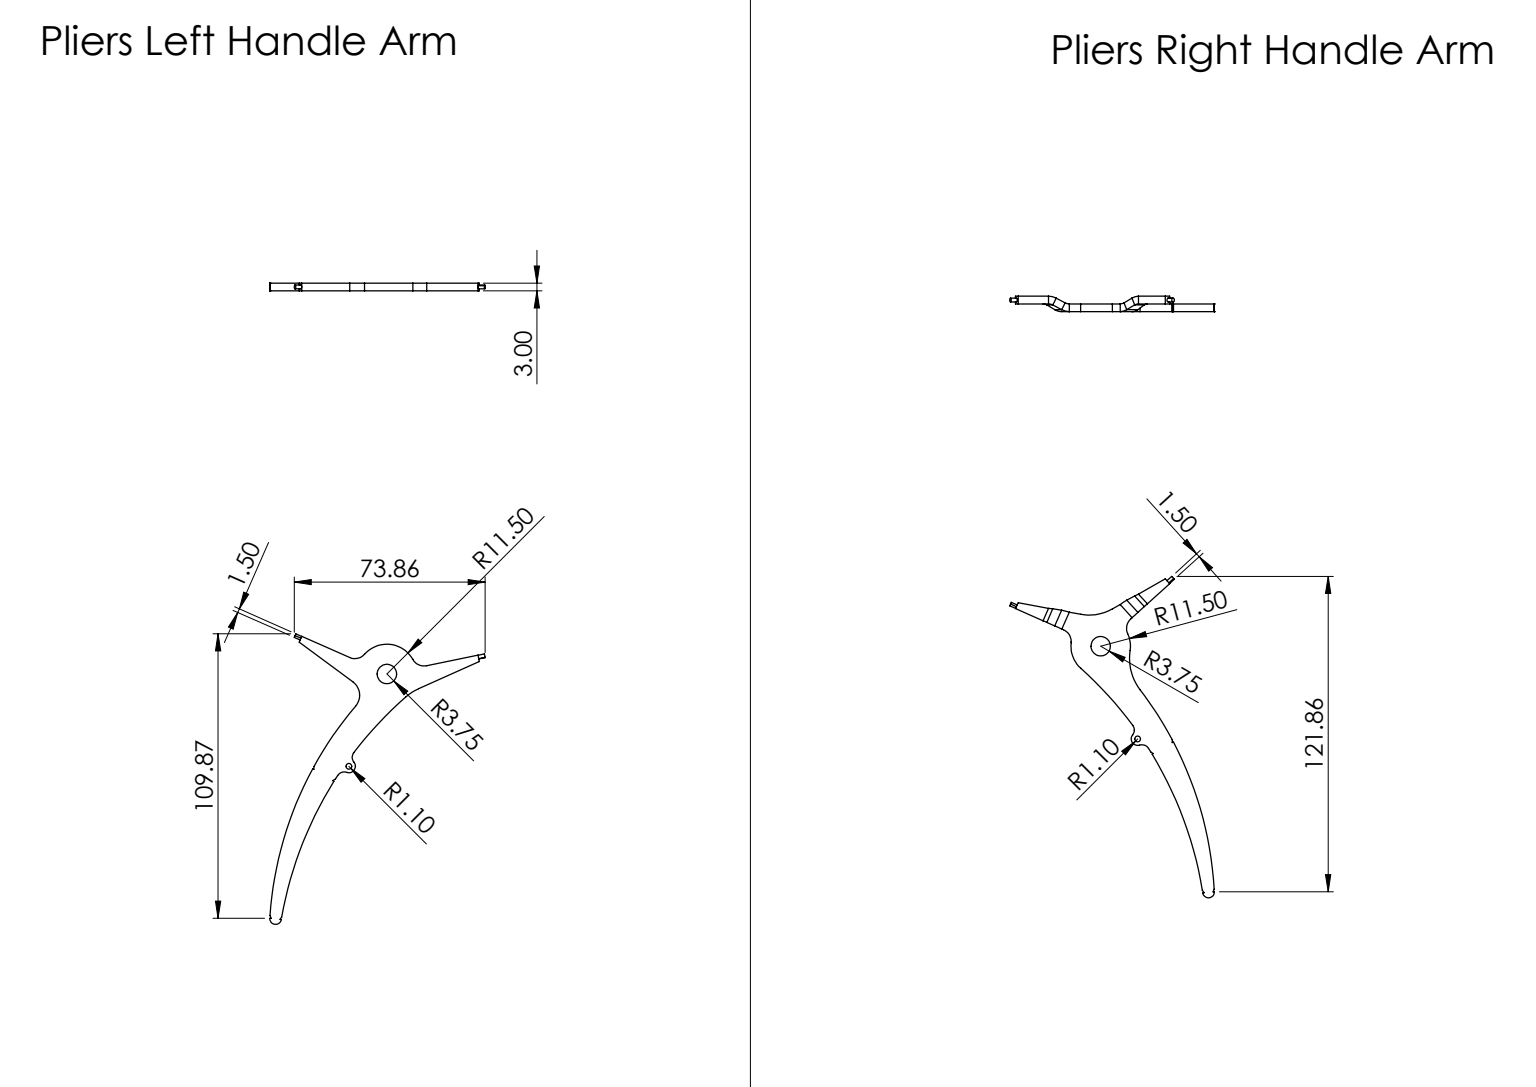
ISO-10303-21;
HEADER;
FILE_DESCRIPTION (('STEP AP214'),
    '1' );
FILE_NAME ('Pliers Right Handle Arm.step',
    '2026-10-09T15:01:35',
    ( '' ),
    ( '' ),
    'SwSTEP 2.0',
    'SolidWorks 2026',
    '' );
FILE_SCHEMA (( 'AUTOMOTIVE_DESIGN' ));
ENDSEC;

DATA;
#2=CIRCLE ( 'NONE', #2039, 3.300000000000002931 ) ;
#5=EDGE_CURVE ( 'NONE', #1930, #3517, #6589, .T. ) ;
#9=CARTESIAN_POINT ( 'NONE',  ( -105.7473861751082040, -118.0666774205683822, -1.188285581044112860E-13 ) ) ;
#10=ORIENTED_EDGE ( 'NONE', *, *, #1499, .F. ) ;
#11=CARTESIAN_POINT ( 'NONE',  ( 39.48483786921892857, -95.33781693134928048, -9.497611030973018842E-14 ) ) ;
#15=EDGE_CURVE ( 'NONE', #320, #2542, #2080, .T. ) ;
#17=CARTESIAN_POINT ( 'NONE',  ( -31.91091272472834817, 16.82560631625344172, 0.006154456448481410852 ) ) ;
#25=AXIS2_PLACEMENT_3D ( 'NONE', #4428, #5501, #4998 ) ;
#26=LINE ( 'NONE', #2324, #1475 ) ;
#28=ADVANCED_FACE ( 'NONE', ( #2146 ), #5063, .T. ) ;
#34=AXIS2_PLACEMENT_3D ( 'NONE', #6184, #972, #7294 ) ;
#35=FACE_OUTER_BOUND ( 'NONE', #4506, .T. ) ;
#37=AXIS2_PLACEMENT_3D ( 'NONE', #1867, #698, #7061 ) ;
#40=AXIS2_PLACEMENT_3D ( 'NONE', #4287, #3708, #845 ) ;
#41=CARTESIAN_POINT ( 'NONE',  ( -7.922926035662746003, 12.41525034409755612, 2.701156757981117984 ) ) ;
#43=FILL_AREA_STYLE_COLOUR ( '', #963 ) ;
#50=AXIS2_PLACEMENT_3D ( 'NONE', #2705, #5732, #561 ) ;
#58=CARTESIAN_POINT ( 'NONE',  ( -15.00216760413269945, 6.625337177075938833, -3.299999999999993161 ) ) ;
#64=CARTESIAN_POINT ( 'NONE',  ( 43.95774332523846795, -95.00278575785266355, -9.454242944073598665E-14 ) ) ;
#68=ADVANCED_FACE ( 'NONE', ( #2687 ), #435, .T. ) ;
#70=VERTEX_POINT ( 'NONE', #2112 ) ;
#75=VERTEX_POINT ( 'NONE', #4424 ) ;
#76=EDGE_CURVE ( 'NONE', #70, #4585, #6096, .T. ) ;
#77=EDGE_CURVE ( 'NONE', #427, #2020, #919, .T. ) ;
#79=CARTESIAN_POINT ( 'NONE',  ( 12.48153656191966476, 18.70005575237079043, -2.479608496603234347 ) ) ;
#81=DIRECTION ( 'NONE',  ( -5.715354789845005112E-18, -9.999836672264339449E-16, 1.000000000000000000 ) ) ;
#89=VERTEX_POINT ( 'NONE', #7308 ) ;
#90=ADVANCED_FACE ( 'NONE', ( #990 ), #3285, .T. ) ;
#92=CARTESIAN_POINT ( 'NONE',  ( 9.769309212388114005, 25.48802373141157673, -2.993845543551514776 ) ) ;
#98=ORIENTED_EDGE ( 'NONE', *, *, #6789, .F. ) ;
#101=PLANE ( 'NONE',  #156 ) ;
#104=EDGE_CURVE ( 'NONE', #5945, #4359, #7121, .T. ) ;
#105=ORIENTED_EDGE ( 'NONE', *, *, #119, .T. ) ;
#106=VERTEX_POINT ( 'NONE', #6746 ) ;
#111=EDGE_CURVE ( 'NONE', #70, #3385, #1232, .T. ) ;
#114=ORIENTED_EDGE ( 'NONE', *, *, #332, .F. ) ;
#117=CARTESIAN_POINT ( 'NONE',  ( -20.16480223318149356, 14.61937842657788345, -2.993845543551524990 ) ) ;
#118=CARTESIAN_POINT ( 'NONE',  ( 9.769309212388092689, 25.48802373141157318, 0.006154456448490518150 ) ) ;
#119=EDGE_CURVE ( 'NONE', #427, #4029, #5685, .T. ) ;
#120=ADVANCED_FACE ( 'NONE', ( #5785 ), #4047, .F. ) ;
#122=AXIS2_PLACEMENT_3D ( 'NONE', #4190, #238, #5631 ) ;
#125=AXIS2_PLACEMENT_3D ( 'NONE', #6895, #3541, #4566 ) ;
#130=ORIENTED_EDGE ( 'NONE', *, *, #2556, .T. ) ;
#138=VERTEX_POINT ( 'NONE', #4690 ) ;
#139=ORIENTED_EDGE ( 'NONE', *, *, #2264, .T. ) ;
#147=CIRCLE ( 'NONE', #6885, 6.299999999999998934 ) ;
#148=AXIS2_PLACEMENT_3D ( 'NONE', #6165, #6059, #1524 ) ;
#150=VECTOR ( 'NONE', #1771, 1000.000000000000227 ) ;
#156=AXIS2_PLACEMENT_3D ( 'NONE', #5801, #629, #4670 ) ;
#161=EDGE_CURVE ( 'NONE', #2317, #4548, #3992, .T. ) ;
#163=LINE ( 'NONE', #7048, #1585 ) ;
#165=CARTESIAN_POINT ( 'NONE',  ( 12.40979888490706706, -30.61452125107581068, 2.999999999999969802 ) ) ;
#174=ORIENTED_EDGE ( 'NONE', *, *, #2963, .T. ) ;
#175=EDGE_CURVE ( 'NONE', #6662, #3589, #2174, .T. ) ;
#178=PLANE ( 'NONE',  #37 ) ;
#184=VERTEX_POINT ( 'NONE', #578 ) ;
#187=CARTESIAN_POINT ( 'NONE',  ( 27.98760434640042050, 26.43260972569849443, -1.493845543551990174 ) ) ;
#190=PLANE ( 'NONE',  #25 ) ;
#191=ORIENTED_EDGE ( 'NONE', *, *, #892, .F. ) ;
#196=PRODUCT ( 'Pliers Right Handle Arm', 'Pliers Right Handle Arm', '', ( #6070 ) ) ;
#198=EDGE_CURVE ( 'NONE', #3368, #5232, #6974, .T. ) ;
#199=ORIENTED_EDGE ( 'NONE', *, *, #978, .F. ) ;
#200=DIRECTION ( 'NONE',  ( 0.9999836672264332815, -0.005715354789844959149, 0.000000000000000000 ) ) ;
#206=EDGE_CURVE ( 'NONE', #2991, #6689, #4958, .T. ) ;
#207=CARTESIAN_POINT ( 'NONE',  ( -17.21006346072928750, 13.86884027412869180, -2.230393353321906247 ) ) ;
#208=ORIENTED_EDGE ( 'NONE', *, *, #252, .F. ) ;
#209=ADVANCED_FACE ( 'NONE', ( #688 ), #379, .F. ) ;
#212=VERTEX_POINT ( 'NONE', #11 ) ;
#213=DIRECTION ( 'NONE',  ( -5.715354789845005112E-18, -9.999836672264339449E-16, 1.000000000000000000 ) ) ;
#216=VERTEX_POINT ( 'NONE', #6910 ) ;
#219=EDGE_LOOP ( 'NONE', ( #5454, #1451, #6530, #3936 ) ) ;
#222=CARTESIAN_POINT ( 'NONE',  ( 27.68174825049008803, -37.24611774345110859, -3.729655473350135253E-14 ) ) ;
#230=DIRECTION ( 'NONE',  ( -0.9999836672264333925, 0.005715354789844960016, 0.000000000000000000 ) ) ;
#233=LINE ( 'NONE', #4722, #5692 ) ;
#238=DIRECTION ( 'NONE',  ( 0.6713653717953971256, -0.7411265327553914206, -1.050567784676125892E-15 ) ) ;
#241=EDGE_LOOP ( 'NONE', ( #2453, #5652, #2656, #1275 ) ) ;
#242=ORIENTED_EDGE ( 'NONE', *, *, #3196, .T. ) ;
#249=ORIENTED_EDGE ( 'NONE', *, *, #5609, .F. ) ;
#250=EDGE_LOOP ( 'NONE', ( #2222, #4590, #6016, #4607 ) ) ;
#251=ORIENTED_EDGE ( 'NONE', *, *, #6437, .T. ) ;
#252=EDGE_CURVE ( 'NONE', #1688, #1547, #147, .T. ) ;
#254=CARTESIAN_POINT ( 'NONE',  ( 23.12979183812720407, 24.32586137474685017, -8.815182418718713109 ) ) ;
#256=FACE_BOUND ( 'NONE', #7433, .T. ) ;
#257=CARTESIAN_POINT ( 'NONE',  ( 12.34225220476766438, -34.27182074065601114, 2.999999999999965805 ) ) ;
#259=ORIENTED_EDGE ( 'NONE', *, *, #1801, .T. ) ;
#260=DIRECTION ( 'NONE',  ( -0.6713653717953970146, 0.7411265327553913096, 7.633377738797892154E-16 ) ) ;
#264=VECTOR ( 'NONE', #2040, 1000.000000000000000 ) ;
#266=CYLINDRICAL_SURFACE ( 'NONE', #6602, 11.50000000000000178 ) ;
#268=ORIENTED_EDGE ( 'NONE', *, *, #1200, .T. ) ;
#269=CIRCLE ( 'NONE', #6408, 140.0000000000000000 ) ;
#271=VECTOR ( 'NONE', #2311, 1000.000000000000000 ) ;
#273=DIRECTION ( 'NONE',  ( -0.4039838799357104993, -0.9147661038495521479, -3.619485620725444841E-16 ) ) ;
#277=AXIS2_PLACEMENT_3D ( 'NONE', #4931, #1502, #1047 ) ;
#280=ORIENTED_EDGE ( 'NONE', *, *, #2225, .T. ) ;
#285=CARTESIAN_POINT ( 'NONE',  ( -15.07233531785332659, 13.90759097395377886, 2.236547809770392803 ) ) ;
#287=VECTOR ( 'NONE', #7438, 1000.000000000000000 ) ;
#288=DIRECTION ( 'NONE',  ( 0.9986925448795970217, 0.05111947575938272093, 5.682652305652042775E-17 ) ) ;
#291=ORIENTED_EDGE ( 'NONE', *, *, #6437, .F. ) ;
#299=PLANE ( 'NONE',  #650 ) ;
#302=ADVANCED_FACE ( 'NONE', ( #3614 ), #3261, .F. ) ;
#305=DIRECTION ( 'NONE',  ( 5.715354789845005112E-18, 9.999836672264339449E-16, -1.000000000000000000 ) ) ;
#307=ORIENTED_EDGE ( 'NONE', *, *, #6778, .T. ) ;
#310=EDGE_CURVE ( 'NONE', #1930, #1079, #233, .T. ) ;
#316=LINE ( 'NONE', #1518, #3268 ) ;
#320=VERTEX_POINT ( 'NONE', #758 ) ;
#321=VERTEX_POINT ( 'NONE', #1855 ) ;
#323=FACE_OUTER_BOUND ( 'NONE', #1179, .T. ) ;
#325=CARTESIAN_POINT ( 'NONE',  ( 6.103722004628568065, 22.16747290800961778, 2.236547809770398576 ) ) ;
#328=ORIENTED_EDGE ( 'NONE', *, *, #1145, .T. ) ;
#331=CARTESIAN_POINT ( 'NONE',  ( -18.51952944085035924, 14.44713361607367830, 0.4060579846639892909 ) ) ;
#332=EDGE_CURVE ( 'NONE', #5680, #3331, #6168, .T. ) ;
#333=LINE ( 'NONE', #6030, #1620 ) ;
#337=FACE_OUTER_BOUND ( 'NONE', #6918, .T. ) ;
#343=EDGE_CURVE ( 'NONE', #1942, #4478, #3077, .T. ) ;
#346=CYLINDRICAL_SURFACE ( 'NONE', #4266, 3.300000000000001599 ) ;
#348=DIRECTION ( 'NONE',  ( -5.715354789845005112E-18, -9.999836672264339449E-16, 1.000000000000000000 ) ) ;
#352=AXIS2_PLACEMENT_3D ( 'NONE', #2407, #3501, #6969 ) ;
#353=ORIENTED_EDGE ( 'NONE', *, *, #3724, .F. ) ;
#356=FACE_OUTER_BOUND ( 'NONE', #779, .T. ) ;
#358=FACE_OUTER_BOUND ( 'NONE', #3624, .T. ) ;
#363=ORIENTED_EDGE ( 'NONE', *, *, #858, .F. ) ;
#373=ORIENTED_EDGE ( 'NONE', *, *, #4079, .F. ) ;
#376=CARTESIAN_POINT ( 'NONE',  ( -18.51952944085035924, 14.44713361607365876, 0.4060579846639944535 ) ) ;
#379=CONICAL_SURFACE ( 'NONE', #3862, 0.7499999999999865663, 1.029744258676651425 ) ;
#381=EDGE_CURVE ( 'NONE', #2927, #5703, #3139, .T. ) ;
#383=VECTOR ( 'NONE', #1135, 1000.000000000000000 ) ;
#385=CARTESIAN_POINT ( 'NONE',  ( 7.541408601728222472, 23.46983215994270822, -2.230393353321886263 ) ) ;
#392=ORIENTED_EDGE ( 'NONE', *, *, #7416, .F. ) ;
#397=AXIS2_PLACEMENT_3D ( 'NONE', #3733, #472, #2723 ) ;
#399=DIRECTION ( 'NONE',  ( -5.715354789845005112E-18, -9.999836672264339449E-16, 1.000000000000000000 ) ) ;
#404=EDGE_CURVE ( 'NONE', #7317, #6686, #1470, .T. ) ;
#410=DIRECTION ( 'NONE',  ( 0.9999836672264332815, -0.005715354789845306094, 0.000000000000000000 ) ) ;
#416=AXIS2_PLACEMENT_3D ( 'NONE', #4573, #2861, #5177 ) ;
#417=AXIS2_PLACEMENT_3D ( 'NONE', #6583, #5829, #3680 ) ;
#418=VERTEX_POINT ( 'NONE', #3343 ) ;
#423=FACE_OUTER_BOUND ( 'NONE', #241, .T. ) ;
#427=VERTEX_POINT ( 'NONE', #5044 ) ;
#434=EDGE_LOOP ( 'NONE', ( #1898, #6648, #1642, #3197 ) ) ;
#435=PLANE ( 'NONE',  #6162 ) ;
#437=DIRECTION ( 'NONE',  ( -0.9999836672264332815, 0.005715354789845002517, 0.000000000000000000 ) ) ;
#438=CARTESIAN_POINT ( 'NONE',  ( 9.018117650298766108, 16.81805756487467107, -0.3999035282154979054 ) ) ;
#444=B_SPLINE_CURVE_WITH_KNOTS ( 'NONE', 1,
 ( #448, #2731 ),
 .UNSPECIFIED., .F., .F.,
 ( 2, 2 ),
 ( 0.000000000000000000, 1.000000000000000000 ),
 .UNSPECIFIED. ) ;
#448=CARTESIAN_POINT ( 'NONE',  ( -20.16480223318149356, 14.61937842657788345, -2.993845543551524990 ) ) ;
#452=FACE_OUTER_BOUND ( 'NONE', #2508, .T. ) ;
#457=CARTESIAN_POINT ( 'NONE',  ( -18.08304078080998778, 14.25436916875867865, -0.4727591279979656558 ) ) ;
#464=LINE ( 'NONE', #4535, #5418 ) ;
#467=ORIENTED_EDGE ( 'NONE', *, *, #4073, .T. ) ;
#468=CARTESIAN_POINT ( 'NONE',  ( -18.51952944085035924, 14.44713361607365876, 0.4060579846639944535 ) ) ;
#472=DIRECTION ( 'NONE',  ( -0.9997217333147506713, -0.02358931830619094214, -2.930269742420907704E-17 ) ) ;
#478=ORIENTED_EDGE ( 'NONE', *, *, #3847, .T. ) ;
#479=EDGE_LOOP ( 'NONE', ( #862, #1759, #191, #5380 ) ) ;
#484=FACE_BOUND ( 'NONE', #3259, .T. ) ;
#488=AXIS2_PLACEMENT_3D ( 'NONE', #3919, #348, #4454 ) ;
#490=EDGE_LOOP ( 'NONE', ( #5569, #3977, #674, #3366 ) ) ;
#491=EDGE_CURVE ( 'NONE', #4550, #2991, #7293, .T. ) ;
#494=DIRECTION ( 'NONE',  ( 0.9999836672264335036, -0.005715354789845041548, 0.000000000000000000 ) ) ;
#497=DIRECTION ( 'NONE',  ( 0.9147661038495522590, -0.4039838799357101107, 0.000000000000000000 ) ) ;
#507=VERTEX_POINT ( 'NONE', #2253 ) ;
#512=VECTOR ( 'NONE', #1190, 1000.000000000000227 ) ;
#516=CYLINDRICAL_SURFACE ( 'NONE', #4587, 147.0000000000000000 ) ;
#518=ORIENTED_EDGE ( 'NONE', *, *, #2225, .F. ) ;
#521=CARTESIAN_POINT ( 'NONE',  ( -12.11759654540111875, 13.15705282150456590, 3.000000000000012879 ) ) ;
#528=AXIS2_PLACEMENT_3D ( 'NONE', #895, #5508, #3787 ) ;
#532=CYLINDRICAL_SURFACE ( 'NONE', #864, 1.100000000000000755 ) ;
#534=CIRCLE ( 'NONE', #4380, 1.100000000000000755 ) ;
#536=EDGE_CURVE ( 'NONE', #5972, #2927, #6293, .T. ) ;
#541=DIRECTION ( 'NONE',  ( -0.005585937530842041351, -0.9773402531220075629, 0.2116006307393995811 ) ) ;
#548=CARTESIAN_POINT ( 'NONE',  ( -20.16480223318149356, 14.61937842657788167, 0.006154456448484012937 ) ) ;
#549=CARTESIAN_POINT ( 'NONE',  ( -32.92087242456759100, 14.53869105662955796, -2.993845543551514776 ) ) ;
#551=CARTESIAN_POINT ( 'NONE',  ( 9.998427761233271482, -32.39925913208585939, -3.252606517456513302E-14 ) ) ;
#552=FACE_OUTER_BOUND ( 'NONE', #4391, .T. ) ;
#553=VERTEX_POINT ( 'NONE', #7278 ) ;
#559=EDGE_LOOP ( 'NONE', ( #876, #3410, #3244, #6024 ) ) ;
#560=DIRECTION ( 'NONE',  ( -5.715354789845005112E-18, -9.999836672264339449E-16, 1.000000000000000000 ) ) ;
#561=DIRECTION ( 'NONE',  ( 0.5894575778543340583, -0.6507077505550991070, -0.4786639607048190914 ) ) ;
#565=ADVANCED_FACE ( 'NONE', ( #742 ), #2725, .T. ) ;
#567=CARTESIAN_POINT ( 'NONE',  ( -11.43300101767539623, 1.239551422827354310, 1.301042606982605321E-15 ) ) ;
#572=CARTESIAN_POINT ( 'NONE',  ( -95.86211798318534250, -102.0316339954322018, -1.027823659516258203E-13 ) ) ;
#573=FACE_OUTER_BOUND ( 'NONE', #2874, .T. ) ;
#576=CARTESIAN_POINT ( 'NONE',  ( -22.27644891976298780, 9.837844043328869859, 3.306154456448478829 ) ) ;
#578=CARTESIAN_POINT ( 'NONE',  ( -15.07233531785332659, 13.90759097395377886, 2.236547809770392803 ) ) ;
#580=ADVANCED_FACE ( 'NONE', ( #3603 ), #190, .T. ) ;
#581=DIRECTION ( 'NONE',  ( -5.715354789845005112E-18, -9.999836672264339449E-16, 1.000000000000000000 ) ) ;
#582=DIRECTION ( 'NONE',  ( -0.7411265327553894222, -0.6713653717953992350, -1.302304562955136501E-15 ) ) ;
#586=ORIENTED_EDGE ( 'NONE', *, *, #2172, .F. ) ;
#588=EDGE_CURVE ( 'NONE', #6745, #5840, #1526, .T. ) ;
#590=CARTESIAN_POINT ( 'NONE',  ( 15.01043771185145381, 6.851040774847843906, 6.938893903907228378E-15 ) ) ;
#595=AXIS2_PLACEMENT_3D ( 'NONE', #4332, #4412, #3266 ) ;
#598=DIRECTION ( 'NONE',  ( -0.6713653717954000122, 0.7411265327553888671, 8.673617379884183383E-16 ) ) ;
#599=AXIS2_PLACEMENT_3D ( 'NONE', #5250, #1318, #2340 ) ;
#600=DIRECTION ( 'NONE',  ( -5.715354789845005112E-18, -9.999836672264339449E-16, 1.000000000000000000 ) ) ;
#601=LINE ( 'NONE', #1580, #3108 ) ;
#602=( NAMED_UNIT ( * ) PLANE_ANGLE_UNIT ( ) SI_UNIT ( $, .RADIAN. ) );
#604=VECTOR ( 'NONE', #6742, 1000.000000000000114 ) ;
#605=FACE_OUTER_BOUND ( 'NONE', #3752, .T. ) ;
#606=CARTESIAN_POINT ( 'NONE',  ( 12.08768627091661330, 18.45115358720316223, -2.230393353321891592 ) ) ;
#609=EDGE_CURVE ( 'NONE', #3815, #7434, #6716, .T. ) ;
#610=DIRECTION ( 'NONE',  ( -0.4702355878038426140, 0.002687607115189603359, -0.8825368370389811146 ) ) ;
#614=AXIS2_PLACEMENT_3D ( 'NONE', #5442, #1438, #2609 ) ;
#621=EDGE_CURVE ( 'NONE', #138, #7431, #5208, .T. ) ;
#622=AXIS2_PLACEMENT_3D ( 'NONE', #58, #5292, #6378 ) ;
#623=ORIENTED_EDGE ( 'NONE', *, *, #2863, .F. ) ;
#624=ORIENTED_EDGE ( 'NONE', *, *, #5316, .T. ) ;
#625=ORIENTED_EDGE ( 'NONE', *, *, #588, .F. ) ;
#627=CIRCLE ( 'NONE', #6512, 5.000000000000000000 ) ;
#629=DIRECTION ( 'NONE',  ( 0.7411265327553895332, 0.6713653717953992350, 1.304512053934558935E-15 ) ) ;
#638=DIRECTION ( 'NONE',  ( 0.6713653717953971256, -0.7411265327553914206, -1.022734129183898348E-15 ) ) ;
#639=CARTESIAN_POINT ( 'NONE',  ( 12.08768627091661330, 18.45115358720316223, -2.230393353321891592 ) ) ;
#640=AXIS2_PLACEMENT_3D ( 'NONE', #2115, #5499, #7276 ) ;
#641=DIRECTION ( 'NONE',  ( -0.3213584079436493934, 0.3547505615521249767, -0.8779981849197497912 ) ) ;
#642=VECTOR ( 'NONE', #2245, 1000.000000000000000 ) ;
#650=AXIS2_PLACEMENT_3D ( 'NONE', #813, #1935, #1504 ) ;
#652=CARTESIAN_POINT ( 'NONE',  ( -11.43300101767539623, 1.239551422827354310, 1.301042606982605321E-15 ) ) ;
#657=ORIENTED_EDGE ( 'NONE', *, *, #1093, .F. ) ;
#659=EDGE_CURVE ( 'NONE', #3712, #5840, #3389, .T. ) ;
#660=VECTOR ( 'NONE', #3819, 1000.000000000000000 ) ;
#661=LINE ( 'NONE', #549, #2800 ) ;
#665=EDGE_LOOP ( 'NONE', ( #2653, #7127, #5002, #3907 ) ) ;
#666=ORIENTED_EDGE ( 'NONE', *, *, #4440, .T. ) ;
#667=ORIENTED_EDGE ( 'NONE', *, *, #161, .T. ) ;
#670=PLANE ( 'NONE',  #2924 ) ;
#674=ORIENTED_EDGE ( 'NONE', *, *, #3234, .T. ) ;
#675=ADVANCED_FACE ( 'NONE', ( #2089 ), #1445, .F. ) ;
#677=LINE ( 'NONE', #2816, #3396 ) ;
#679=DIRECTION ( 'NONE',  ( -0.7411265327553895332, -0.6713653717953993461, -1.302304562955136699E-15 ) ) ;
#682=DIRECTION ( 'NONE',  ( -0.6713653717954000122, 0.7411265327553888671, 8.673617379884183383E-16 ) ) ;
#686=DIRECTION ( 'NONE',  ( 0.9999836672264335036, -0.005715354789845041548, 0.000000000000000000 ) ) ;
#687=ORIENTED_EDGE ( 'NONE', *, *, #4816, .T. ) ;
#688=FACE_OUTER_BOUND ( 'NONE', #4920, .T. ) ;
#689=CARTESIAN_POINT ( 'NONE',  ( 3.749938752099124972, -0.02143258046191576227, 0.000000000000000000 ) ) ;
#694=ADVANCED_FACE ( 'NONE', ( #3779 ), #3812, .F. ) ;
#697=FACE_OUTER_BOUND ( 'NONE', #6983, .T. ) ;
#698=DIRECTION ( 'NONE',  ( -3.872980802086269402E-16, 2.250611045722691657E-16, -1.000000000000000000 ) ) ;
#700=DIRECTION ( 'NONE',  ( -5.715354789845005112E-18, -9.999836672264339449E-16, 1.000000000000000000 ) ) ;
#702=LINE ( 'NONE', #6543, #3867 ) ;
#710=CARTESIAN_POINT ( 'NONE',  ( -19.14099990134980089, 14.35202449503593058, -2.928563623636439850 ) ) ;
#714=EDGE_CURVE ( 'NONE', #1079, #216, #5791, .T. ) ;
#719=B_SPLINE_CURVE_WITH_KNOTS ( 'NONE', 1,
 ( #5205, #1695 ),
 .UNSPECIFIED., .F., .F.,
 ( 2, 2 ),
 ( 0.000000000000000000, 1.000000000000000000 ),
 .UNSPECIFIED. ) ;
#720=DIRECTION ( 'NONE',  ( -0.8481698128690331462, 0.5297244269785085224, 5.248681837068071230E-16 ) ) ;
#722=UNCERTAINTY_MEASURE_WITH_UNIT (LENGTH_MEASURE( 1.000000000000000082E-05 ), #4037, 'distance_accuracy_value', 'NONE');
#727=ORIENTED_EDGE ( 'NONE', *, *, #7316, .T. ) ;
#728=ORIENTED_EDGE ( 'NONE', *, *, #5712, .F. ) ;
#733=CARTESIAN_POINT ( 'NONE',  ( 25.86911032031090940, 23.43408864831972238, -6.178731080732846159 ) ) ;
#735=EDGE_LOOP ( 'NONE', ( #7209, #6312, #4963, #4617 ) ) ;
#736=VECTOR ( 'NONE', #1817, 1000.000000000000000 ) ;
#740=DIRECTION ( 'NONE',  ( -5.715354789845005112E-18, -9.999836672264339449E-16, 1.000000000000000000 ) ) ;
#742=FACE_OUTER_BOUND ( 'NONE', #988, .T. ) ;
#749=EDGE_CURVE ( 'NONE', #6942, #4841, #1471, .T. ) ;
#751=AXIS2_PLACEMENT_3D ( 'NONE', #5959, #3597, #6467 ) ;
#755=VECTOR ( 'NONE', #3723, 1000.000000000000227 ) ;
#758=CARTESIAN_POINT ( 'NONE',  ( 28.12455780688317475, -37.01391159201033076, 2.999999999999963141 ) ) ;
#760=VECTOR ( 'NONE', #5141, 1000.000000000000000 ) ;
#770=ORIENTED_EDGE ( 'NONE', *, *, #978, .T. ) ;
#772=ORIENTED_EDGE ( 'NONE', *, *, #2683, .F. ) ;
#775=CARTESIAN_POINT ( 'NONE',  ( -13.14279338728291080, 13.42477640308646514, 3.000000000000013323 ) ) ;
#778=ORIENTED_EDGE ( 'NONE', *, *, #5101, .T. ) ;
#779=EDGE_LOOP ( 'NONE', ( #7399, #930, #4175, #7407 ) ) ;
#790=CARTESIAN_POINT ( 'NONE',  ( -32.59768532061891477, 15.27050393970957565, -0.7438455435515303193 ) ) ;
#793=ADVANCED_FACE ( 'NONE', ( #5721 ), #6794, .F. ) ;
#796=CARTESIAN_POINT ( 'NONE',  ( 3.749938752099124972, -0.02143258046191576227, 0.000000000000000000 ) ) ;
#800=DIRECTION ( 'NONE',  ( -0.9147661038495522590, 0.4039838799357101107, 0.000000000000000000 ) ) ;
#804=ORIENTED_EDGE ( 'NONE', *, *, #971, .F. ) ;
#809=EDGE_LOOP ( 'NONE', ( #5426, #6635, #3694, #2758 ) ) ;
#810=ORIENTED_EDGE ( 'NONE', *, *, #2697, .F. ) ;
#811=DIRECTION ( 'NONE',  ( 5.715354789845005112E-18, 9.999836672264339449E-16, -1.000000000000000000 ) ) ;
#813=CARTESIAN_POINT ( 'NONE',  ( -16.17971834312690760, 1.679495322419672920, 0.9550319896483219217 ) ) ;
#826=LINE ( 'NONE', #796, #7371 ) ;
#827=EDGE_CURVE ( 'NONE', #7060, #7093, #4582, .T. ) ;
#830=PLANE ( 'NONE',  #614 ) ;
#831=ORIENTED_EDGE ( 'NONE', *, *, #4632, .T. ) ;
#832=ORIENTED_EDGE ( 'NONE', *, *, #4592, .F. ) ;
#840=AXIS2_PLACEMENT_3D ( 'NONE', #4513, #4429, #7314 ) ;
#841=EDGE_LOOP ( 'NONE', ( #6668, #2509, #3147, #2037 ) ) ;
#842=ORIENTED_EDGE ( 'NONE', *, *, #1448, .F. ) ;
#843=ORIENTED_EDGE ( 'NONE', *, *, #5006, .F. ) ;
#845=DIRECTION ( 'NONE',  ( 5.715354789845005112E-18, 9.999836672264339449E-16, -1.000000000000000000 ) ) ;
#848=CARTESIAN_POINT ( 'NONE',  ( 39.48483786921892857, -95.33781693134928048, 2.999999999999904965 ) ) ;
#856=DIRECTION ( 'NONE',  ( 0.4644123028815776988, -0.8856191127862077517, -8.829503670900357056E-16 ) ) ;
#857=VECTOR ( 'NONE', #5182, 1000.000000000000227 ) ;
#858=EDGE_CURVE ( 'NONE', #4757, #5242, #6486, .T. ) ;
#862=ORIENTED_EDGE ( 'NONE', *, *, #1392, .T. ) ;
#864=AXIS2_PLACEMENT_3D ( 'NONE', #2929, #2850, #6848 ) ;
#867=LINE ( 'NONE', #3121, #7137 ) ;
#872=CIRCLE ( 'NONE', #1358, 2.999999999999999556 ) ;
#876=ORIENTED_EDGE ( 'NONE', *, *, #1819, .T. ) ;
#882=CIRCLE ( 'NONE', #5955, 147.0000000000000000 ) ;
#886=DIRECTION ( 'NONE',  ( 0.6713653717953965705, -0.7411265327553918647, -7.095217611944926095E-16 ) ) ;
#889=AXIS2_PLACEMENT_3D ( 'NONE', #6367, #5354, #2966 ) ;
#890=ORIENTED_EDGE ( 'NONE', *, *, #5, .F. ) ;
#891=EDGE_LOOP ( 'NONE', ( #5274, #7034, #3632, #1068 ) ) ;
#892=EDGE_CURVE ( 'NONE', #5232, #3517, #2314, .T. ) ;
#893=ADVANCED_FACE ( 'NONE', ( #423 ), #3307, .T. ) ;
#895=CARTESIAN_POINT ( 'NONE',  ( -17.18648583462957902, 1.679248046991888677, -3.299999999999998046 ) ) ;
#899=ORIENTED_EDGE ( 'NONE', *, *, #5637, .F. ) ;
#900=ORIENTED_EDGE ( 'NONE', *, *, #1718, .F. ) ;
#901=VERTEX_POINT ( 'NONE', #4675 ) ;
#902=ADVANCED_FACE ( 'NONE', ( #5809 ), #5168, .T. ) ;
#909=VERTEX_POINT ( 'NONE', #6889 ) ;
#912=FACE_OUTER_BOUND ( 'NONE', #841, .T. ) ;
#917=CARTESIAN_POINT ( 'NONE',  ( -34.88460058024264043, 16.28046363954882736, -1.493845543551999944 ) ) ;
#918=EDGE_LOOP ( 'NONE', ( #5155, #6456, #1274, #4233 ) ) ;
#919=LINE ( 'NONE', #1633, #2892 ) ;
#920=ORIENTED_EDGE ( 'NONE', *, *, #714, .T. ) ;
#924=CARTESIAN_POINT ( 'NONE',  ( 1.714606436953501688E-17, 2.999951001679301835E-15, 0.000000000000000000 ) ) ;
#928=ORIENTED_EDGE ( 'NONE', *, *, #659, .F. ) ;
#929=EDGE_LOOP ( 'NONE', ( #2961, #1882, #6390, #623 ) ) ;
#930=ORIENTED_EDGE ( 'NONE', *, *, #6257, .T. ) ;
#931=CARTESIAN_POINT ( 'NONE',  ( -17.21006346072928750, 13.86884027412869180, -2.230393353321906247 ) ) ;
#935=EDGE_CURVE ( 'NONE', #2431, #6755, #5853, .T. ) ;
#938=ORIENTED_EDGE ( 'NONE', *, *, #6081, .T. ) ;
#947=FACE_OUTER_BOUND ( 'NONE', #2701, .T. ) ;
#950=DIRECTION ( 'NONE',  ( -0.4039838799357112764, -0.9147661038495517039, -1.194615830541411051E-15 ) ) ;
#953=DIRECTION ( 'NONE',  ( -5.715354789845005112E-18, -9.999836672264339449E-16, 1.000000000000000000 ) ) ;
#956=LINE ( 'NONE', #4314, #4970 ) ;
#962=ORIENTED_EDGE ( 'NONE', *, *, #1280, .T. ) ;
#963=COLOUR_RGB ( '', 0.31764706, 0.68627451, 0.89019608) ;
#966=FACE_OUTER_BOUND ( 'NONE', #5767, .T. ) ;
#971=EDGE_CURVE ( 'NONE', #7093, #6135, #4708, .T. ) ;
#972=DIRECTION ( 'NONE',  ( 0.1845982795403117716, 0.9828140593167952188, 9.838530518984746718E-16 ) ) ;
#976=AXIS2_PLACEMENT_3D ( 'NONE', #3320, #6787, #3923 ) ;
#978=EDGE_CURVE ( 'NONE', #3496, #75, #3836, .T. ) ;
#980=AXIS2_PLACEMENT_3D ( 'NONE', #2792, #4661, #4049 ) ;
#981=VECTOR ( 'NONE', #886, 1000.000000000000114 ) ;
#988=EDGE_LOOP ( 'NONE', ( #727, #6330, #1513, #4803 ) ) ;
#990=FACE_OUTER_BOUND ( 'NONE', #1162, .T. ) ;
#991=ADVANCED_FACE ( 'NONE', ( #5202 ), #532, .F. ) ;
#993=CIRCLE ( 'NONE', #6523, 2.500000000000000000 ) ;
#998=DIRECTION ( 'NONE',  ( 0.9999836672264333925, -0.005715354789844388425, 0.000000000000000000 ) ) ;
#1000=VERTEX_POINT ( 'NONE', #6366 ) ;
#1011=DIRECTION ( 'NONE',  ( -0.005715354789845003385, -0.9999836672264335036, -1.000000000000000472E-15 ) ) ;
#1015=CIRCLE ( 'NONE', #3763, 147.0000000000000000 ) ;
#1026=B_SPLINE_CURVE_WITH_KNOTS ( 'NONE', 3,
 ( #6744, #3958, #2717, #1593 ),
 .UNSPECIFIED., .F., .F.,
 ( 4, 4 ),
 ( 0.000000000000000000, 1.000000000000000000 ),
 .UNSPECIFIED. ) ;
#1034=CARTESIAN_POINT ( 'NONE',  ( -12.11759654540111875, 13.15705282150456945, 1.301042606982605321E-14 ) ) ;
#1039=CARTESIAN_POINT ( 'NONE',  ( 12.15447797363371052, 11.01039466689934798, -3.299999999999988720 ) ) ;
#1042=ORIENTED_EDGE ( 'NONE', *, *, #5917, .T. ) ;
#1046=EDGE_LOOP ( 'NONE', ( #6190, #5981, #4892, #6244 ) ) ;
#1047=DIRECTION ( 'NONE',  ( 0.9999836672264333925, -0.005715354789844381486, 0.000000000000000000 ) ) ;
#1048=ORIENTED_EDGE ( 'NONE', *, *, #3659, .F. ) ;
#1050=DIRECTION ( 'NONE',  ( 0.9999836672264335036, -0.005715354789845041548, 0.000000000000000000 ) ) ;
#1052=ORIENTED_EDGE ( 'NONE', *, *, #2646, .F. ) ;
#1053=EDGE_CURVE ( 'NONE', #507, #3368, #677, .T. ) ;
#1054=ORIENTED_EDGE ( 'NONE', *, *, #3325, .F. ) ;
#1062=ORIENTED_EDGE ( 'NONE', *, *, #621, .F. ) ;
#1064=CARTESIAN_POINT ( 'NONE',  ( 43.95483829995806957, -94.87490738911687060, 2.999999999999905409 ) ) ;
#1065=CYLINDRICAL_SURFACE ( 'NONE', #6259, 17.99999999999999645 ) ;
#1068=ORIENTED_EDGE ( 'NONE', *, *, #5637, .T. ) ;
#1069=DIRECTION ( 'NONE',  ( -5.715354789845005112E-18, -9.999836672264339449E-16, 1.000000000000000000 ) ) ;
#1071=EDGE_CURVE ( 'NONE', #3368, #3946, #5330, .T. ) ;
#1072=CARTESIAN_POINT ( 'NONE',  ( 27.68174825049008803, -37.24611774345110859, 2.999999999999962697 ) ) ;
#1073=PLANE ( 'NONE',  #1248 ) ;
#1078=ORIENTED_EDGE ( 'NONE', *, *, #3929, .T. ) ;
#1079=VERTEX_POINT ( 'NONE', #6501 ) ;
#1085=FACE_OUTER_BOUND ( 'NONE', #5107, .T. ) ;
#1086=PLANE ( 'NONE',  #50 ) ;
#1090=AXIS2_PLACEMENT_3D ( 'NONE', #4036, #2774, #6774 ) ;
#1093=EDGE_CURVE ( 'NONE', #184, #3517, #4210, .T. ) ;
#1094=DIRECTION ( 'NONE',  ( 5.715354789845005112E-18, 9.999836672264339449E-16, -1.000000000000000000 ) ) ;
#1096=CARTESIAN_POINT ( 'NONE',  ( -34.88460058024264043, 16.28046363954882736, -1.493845543551999944 ) ) ;
#1099=ORIENTED_EDGE ( 'NONE', *, *, #1810, .F. ) ;
#1102=DIRECTION ( 'NONE',  ( 0.9999836672264332815, -0.005715354789845002517, 0.000000000000000000 ) ) ;
#1103=CARTESIAN_POINT ( 'NONE',  ( -32.59768532061886503, 15.27050393970963782, -2.243845543551999722 ) ) ;
#1106=CARTESIAN_POINT ( 'NONE',  ( 3.875821393968650330, 20.14928133654075282, 2.038300084272748336E-14 ) ) ;
#1110=CARTESIAN_POINT ( 'NONE',  ( -15.00216760413269945, 6.625337177075933504, 3.000000000000006661 ) ) ;
#1112=DIRECTION ( 'NONE',  ( 0.9147661038495522590, -0.4039838799357101107, 0.000000000000000000 ) ) ;
#1115=DIRECTION ( 'NONE',  ( -0.7411265327553938631, -0.6713653717953943501, -6.570922257487907035E-16 ) ) ;
#1120=ORIENTED_EDGE ( 'NONE', *, *, #2536, .F. ) ;
#1125=DIRECTION ( 'NONE',  ( 5.715354789845005112E-18, 9.999836672264339449E-16, -1.000000000000000000 ) ) ;
#1129=AXIS2_PLACEMENT_3D ( 'NONE', #5439, #273, #3766 ) ;
#1133=ORIENTED_EDGE ( 'NONE', *, *, #6582, .T. ) ;
#1135=DIRECTION ( 'NONE',  ( -0.1937640608316276714, 0.9810481582114290999, 9.799247046208297627E-16 ) ) ;
#1136=DIRECTION ( 'NONE',  ( -0.9147661038495505936, 0.4039838799357137744, 3.987490689252539707E-16 ) ) ;
#1138=CARTESIAN_POINT ( 'NONE',  ( 14.19688052452437255, 19.82243459985110334, -2.993845543551514776 ) ) ;
#1141=CARTESIAN_POINT ( 'NONE',  ( -20.16480223318149356, 14.61937842657788345, -2.993845543551524990 ) ) ;
#1144=EDGE_CURVE ( 'NONE', #909, #3946, #702, .T. ) ;
#1145=EDGE_CURVE ( 'NONE', #5783, #2991, #872, .T. ) ;
#1146=ORIENTED_EDGE ( 'NONE', *, *, #3847, .F. ) ;
#1147=CIRCLE ( 'NONE', #5355, 0.7500000000000000000 ) ;
#1148=CARTESIAN_POINT ( 'NONE',  ( -7.672523287152989369, -8.566351989504941145, 2.999999999999991562 ) ) ;
#1150=CARTESIAN_POINT ( 'NONE',  ( 26.82878048574519525, 24.30342645899339971, 2.428612866367529932E-14 ) ) ;
#1154=ORIENTED_EDGE ( 'NONE', *, *, #5518, .F. ) ;
#1155=CARTESIAN_POINT ( 'NONE',  ( 31.14423615379030608, -4.720863734206126594, -4.336808689942017736E-15 ) ) ;
#1156=DIRECTION ( 'NONE',  ( -0.8039121061460990925, 0.3550279469270785637, -0.4771587602596087385 ) ) ;
#1157=CARTESIAN_POINT ( 'NONE',  ( -24.22739558392570203, 5.420192826457481239, 3.306154456448477497 ) ) ;
#1162=EDGE_LOOP ( 'NONE', ( #4430, #5001, #2658, #3993 ) ) ;
#1165=DIRECTION ( 'NONE',  ( 0.7411265327553913096, 0.6713653717953970146, 6.200790563844063010E-16 ) ) ;
#1170=VERTEX_POINT ( 'NONE', #4747 ) ;
#1171=ORIENTED_EDGE ( 'NONE', *, *, #1304, .F. ) ;
#1174=ADVANCED_FACE ( 'NONE', ( #2548 ), #6577, .T. ) ;
#1175=DIRECTION ( 'NONE',  ( 0.9147661038495520369, -0.4039838799357104437, -3.987490689252506674E-16 ) ) ;
#1176=DIRECTION ( 'NONE',  ( -0.3213584079436493934, 0.3547505615521249767, -0.8779981849197497912 ) ) ;
#1179=EDGE_LOOP ( 'NONE', ( #1416, #4551, #7282, #4937 ) ) ;
#1183=LINE ( 'NONE', #7383, #760 ) ;
#1190=DIRECTION ( 'NONE',  ( -0.1248576012279878633, 0.9921746718272910215, 1.096417580487672448E-15 ) ) ;
#1192=DIRECTION ( 'NONE',  ( -0.3963837160139272453, -0.9180849359830441925, -9.203354146796070219E-16 ) ) ;
#1196=EDGE_LOOP ( 'NONE', ( #6566, #5335, #307, #6567 ) ) ;
#1199=CARTESIAN_POINT ( 'NONE',  ( 13.19545720709724890, -35.82600185752891520, 2.999999999999964473 ) ) ;
#1200=EDGE_CURVE ( 'NONE', #5032, #2317, #7140, .T. ) ;
#1201=DIRECTION ( 'NONE',  ( 0.7411265327553913096, 0.6713653717953970146, 6.200790563844063010E-16 ) ) ;
#1206=ORIENTED_EDGE ( 'NONE', *, *, #104, .F. ) ;
#1208=CARTESIAN_POINT ( 'NONE',  ( 14.38237858429363492, 13.02858623836822005, 2.236547809770392359 ) ) ;
#1209=CARTESIAN_POINT ( 'NONE',  ( 19.86817077757012484, -41.71399671145084653, -4.163336342344337027E-14 ) ) ;
#1210=CARTESIAN_POINT ( 'NONE',  ( -7.741417275248890562, 12.33509147838778475, 3.000000000000011990 ) ) ;
#1214=ORIENTED_EDGE ( 'NONE', *, *, #2963, .F. ) ;
#1215=ORIENTED_EDGE ( 'NONE', *, *, #111, .T. ) ;
#1216=ADVANCED_FACE ( 'NONE', ( #1976 ), #1836, .F. ) ;
#1218=CARTESIAN_POINT ( 'NONE',  ( -28.32684271132278298, 12.56450996214383409, -1.493845543551522104 ) ) ;
#1224=ADVANCED_FACE ( 'NONE', ( #4142 ), #6440, .T. ) ;
#1232=CIRCLE ( 'NONE', #976, 1.100000000000000755 ) ;
#1233=EDGE_LOOP ( 'NONE', ( #3225, #3020, #728, #6540 ) ) ;
#1234=ADVANCED_FACE ( 'NONE', ( #3745 ), #5983, .T. ) ;
#1237=DIRECTION ( 'NONE',  ( 1.046706025223848628E-16, -1.111638688234981404E-15, 1.000000000000000000 ) ) ;
#1248=AXIS2_PLACEMENT_3D ( 'NONE', #5184, #2307, #5150 ) ;
#1250=AXIS2_PLACEMENT_3D ( 'NONE', #254, #2589, #1387 ) ;
#1253=VECTOR ( 'NONE', #3013, 1000.000000000000000 ) ;
#1257=CONICAL_SURFACE ( 'NONE', #2569, 0.7499999999999872324, 1.029744258676647872 ) ;
#1261=LINE ( 'NONE', #1150, #3487 ) ;
#1265=ORIENTED_EDGE ( 'NONE', *, *, #6853, .T. ) ;
#1266=DIRECTION ( 'NONE',  ( 5.715354789845005112E-18, 9.999836672264339449E-16, -1.000000000000000000 ) ) ;
#1267=CIRCLE ( 'NONE', #2579, 3.750000000000000000 ) ;
#1272=LINE ( 'NONE', #3552, #4709 ) ;
#1274=ORIENTED_EDGE ( 'NONE', *, *, #4073, .F. ) ;
#1275=ORIENTED_EDGE ( 'NONE', *, *, #7010, .F. ) ;
#1277=CARTESIAN_POINT ( 'NONE',  ( 18.04796579205319063, 16.34913706177017900, -2.993845543551523214 ) ) ;
#1280=EDGE_CURVE ( 'NONE', #2431, #1079, #3183, .T. ) ;
#1281=EDGE_CURVE ( 'NONE', #3216, #6745, #5458, .T. ) ;
#1285=CARTESIAN_POINT ( 'NONE',  ( 14.29543924104632779, -35.83228874779774742, -3.556183125752454544E-14 ) ) ;
#1286=ADVANCED_FACE ( 'NONE', ( #3299 ), #1611, .F. ) ;
#1288=DIRECTION ( 'NONE',  ( -0.8748844214391259255, 0.1369338178966306718, -0.4645711771509057897 ) ) ;
#1293=CARTESIAN_POINT ( 'NONE',  ( 18.04796579205319063, 16.34913706177017900, -2.993845543551572952 ) ) ;
#1295=ORIENTED_EDGE ( 'NONE', *, *, #5654, .T. ) ;
#1300=DIRECTION ( 'NONE',  ( -0.4039838799357108323, -0.9147661038495518149, -9.170600743851223106E-16 ) ) ;
#1302=ORIENTED_EDGE ( 'NONE', *, *, #536, .F. ) ;
#1303=ORIENTED_EDGE ( 'NONE', *, *, #3724, .T. ) ;
#1304=EDGE_CURVE ( 'NONE', #89, #4550, #2438, .T. ) ;
#1307=DIRECTION ( 'NONE',  ( -5.715354789845005112E-18, -9.999836672264339449E-16, 1.000000000000000000 ) ) ;
#1310=EDGE_LOOP ( 'NONE', ( #6388, #5982, #1827, #6956 ) ) ;
#1311=ORIENTED_EDGE ( 'NONE', *, *, #111, .F. ) ;
#1313=ADVANCED_FACE ( 'NONE', ( #2049 ), #6174, .F. ) ;
#1318=DIRECTION ( 'NONE',  ( -5.715354789845005112E-18, -9.999836672264339449E-16, 1.000000000000000000 ) ) ;
#1320=VECTOR ( 'NONE', #1880, 1000.000000000000000 ) ;
#1323=CARTESIAN_POINT ( 'NONE',  ( -34.88460058024264043, 16.28046363954882736, -1.493845543551999944 ) ) ;
#1324=LINE ( 'NONE', #652, #1320 ) ;
#1337=ORIENTED_EDGE ( 'NONE', *, *, #6426, .F. ) ;
#1340=FACE_OUTER_BOUND ( 'NONE', #6786, .T. ) ;
#1341=CARTESIAN_POINT ( 'NONE',  ( -28.02385480137132845, 13.25058454003066188, -1.493845543551522104 ) ) ;
#1347=( NAMED_UNIT ( * ) PLANE_ANGLE_UNIT ( ) SI_UNIT ( $, .RADIAN. ) );
#1351=EDGE_CURVE ( 'NONE', #106, #6538, #6419, .T. ) ;
#1358=AXIS2_PLACEMENT_3D ( 'NONE', #3102, #811, #5464 ) ;
#1365=VECTOR ( 'NONE', #582, 1000.000000000000227 ) ;
#1369=DIRECTION ( 'NONE',  ( 0.9999836672264332815, -0.005715354789847320975, 0.000000000000000000 ) ) ;
#1375=DIRECTION ( 'NONE',  ( 1.046706025223848628E-16, -1.111638688234981404E-15, 1.000000000000000000 ) ) ;
#1376=CARTESIAN_POINT ( 'NONE',  ( 26.67188031194815068, 24.16129507000589172, 0.006154456448489217107 ) ) ;
#1377=VERTEX_POINT ( 'NONE', #5615 ) ;
#1378=ORIENTED_EDGE ( 'NONE', *, *, #5609, .T. ) ;
#1381=DIRECTION ( 'NONE',  ( 0.6713653717953966815, -0.7411265327553919757, -7.372773368101216216E-16 ) ) ;
#1387=DIRECTION ( 'NONE',  ( -0.1950386857152336950, 0.001114733493296387375, 0.9807949166078060443 ) ) ;
#1388=CARTESIAN_POINT ( 'NONE',  ( -31.91091272472834817, 16.82560631625344172, -2.993845543551523214 ) ) ;
#1391=ORIENTED_EDGE ( 'NONE', *, *, #1587, .F. ) ;
#1392=EDGE_CURVE ( 'NONE', #4056, #1930, #444, .T. ) ;
#1395=CARTESIAN_POINT ( 'NONE',  ( 10.07902270299396008, 17.77910117033601978, 2.236547809770398132 ) ) ;
#1397=B_SPLINE_SURFACE_WITH_KNOTS ( 'NONE', 1, 3, ( 
 ( #1558, #3846, #1489, #2614 ),
 ( #6603, #7205, #4350, #438 ) ),
 .UNSPECIFIED., .F., .F., .F.,
 ( 2, 2 ),
 ( 4, 4 ),
 ( 0.000000000000000000, 1.000000000000000000 ),
 ( 0.000000000000000000, 1.000000000000000000 ),
 .UNSPECIFIED. ) ;
#1398=EDGE_LOOP ( 'NONE', ( #6951, #3861 ) ) ;
#1400=EDGE_CURVE ( 'NONE', #1506, #4731, #5036, .T. ) ;
#1411=CARTESIAN_POINT ( 'NONE',  ( 24.99346688245966419, 26.01411140189437532, -2.993845543551503674 ) ) ;
#1416=ORIENTED_EDGE ( 'NONE', *, *, #2598, .F. ) ;
#1425=DIRECTION ( 'NONE',  ( -5.715354789845005112E-18, -9.999836672264339449E-16, 1.000000000000000000 ) ) ;
#1427=EDGE_CURVE ( 'NONE', #1688, #4757, #4669, .T. ) ;
#1428=ORIENTED_EDGE ( 'NONE', *, *, #6641, .F. ) ;
#1434=FACE_OUTER_BOUND ( 'NONE', #2612, .T. ) ;
#1438=DIRECTION ( 'NONE',  ( 0.6713653717953944611, -0.7411265327553937521, 8.447904732807262513E-16 ) ) ;
#1441=VERTEX_POINT ( 'NONE', #6801 ) ;
#1442=CARTESIAN_POINT ( 'NONE',  ( 24.19069689082242647, 25.28690498020820243, -6.178731080732834613 ) ) ;
#1445=CYLINDRICAL_SURFACE ( 'NONE', #2310, 3.750000000000000000 ) ;
#1448=EDGE_CURVE ( 'NONE', #1686, #3666, #1762, .T. ) ;
#1449=VECTOR ( 'NONE', #7161, 999.9999999999998863 ) ;
#1451=ORIENTED_EDGE ( 'NONE', *, *, #6294, .T. ) ;
#1454=CARTESIAN_POINT ( 'NONE',  ( 1.714606436953501688E-17, 2.999951001679301835E-15, 0.000000000000000000 ) ) ;
#1458=EDGE_CURVE ( 'NONE', #184, #5486, #2499, .T. ) ;
#1460=CLOSED_SHELL ( 'NONE', ( #7301, #5880, #2345, #2597, #6498, #6069, #2274, #991, #793, #565, #6071, #6863, #28, #7063, #7051, #902, #68, #6364, #7274, #4952, #6466, #4312, #2583, #1884, #4344, #90, #7432, #4953, #1286, #1224, #6473, #120, #3830, #694, #675, #2964, #6380, #5833, #3888, #1660, #5476, #7096, #4922, #5187, #5314, #7336, #2375, #4215, #4756, #1174, #6875, #893, #1708, #3548, #1313, #5366, #6201, #2864, #2545, #6013, #2757, #1234, #3130, #580, #1996, #6570, #3419, #3564, #5517, #7234, #3002, #6975, #5879, #1216, #4911, #2918, #2493 ) ) ;
#1461=DIRECTION ( 'NONE',  ( 1.850371707708594760E-14, 4.625929269271487058E-14, -1.000000000000000000 ) ) ;
#1463=EDGE_LOOP ( 'NONE', ( #6688, #2595 ) ) ;
#1465=VECTOR ( 'NONE', #6169, 1000.000000000000000 ) ;
#1468=VERTEX_POINT ( 'NONE', #1795 ) ;
#1469=AXIS2_PLACEMENT_3D ( 'NONE', #7107, #2561, #5617 ) ;
#1470=B_SPLINE_CURVE_WITH_KNOTS ( 'NONE', 3,
 ( #2814, #2848, #5693, #1576 ),
 .UNSPECIFIED., .F., .F.,
 ( 4, 4 ),
 ( 0.000000000000000000, 1.000000000000000000 ),
 .UNSPECIFIED. ) ;
#1471=CIRCLE ( 'NONE', #6892, 3.299999999999999378 ) ;
#1472=AXIS2_PLACEMENT_3D ( 'NONE', #6296, #638, #3948 ) ;
#1475=VECTOR ( 'NONE', #4637, 1000.000000000000114 ) ;
#1485=VECTOR ( 'NONE', #4544, 1000.000000000000000 ) ;
#1487=CIRCLE ( 'NONE', #416, 5.000000000000000000 ) ;
#1489=CARTESIAN_POINT ( 'NONE',  ( 9.290270525626649345, 17.28063226168697497, 2.735643510310428628 ) ) ;
#1494=ORIENTED_EDGE ( 'NONE', *, *, #6459, .T. ) ;
#1495=VECTOR ( 'NONE', #5438, 1000.000000000000227 ) ;
#1499=EDGE_CURVE ( 'NONE', #2710, #3657, #4057, .T. ) ;
#1502=DIRECTION ( 'NONE',  ( 5.715354789845005112E-18, 9.999836672264339449E-16, -1.000000000000000000 ) ) ;
#1504=DIRECTION ( 'NONE',  ( -0.005585937530842041351, -0.9773402531220075629, 0.2116006307393995811 ) ) ;
#1506=VERTEX_POINT ( 'NONE', #5159 ) ;
#1512=LINE ( 'NONE', #6623, #4455 ) ;
#1513=ORIENTED_EDGE ( 'NONE', *, *, #6544, .F. ) ;
#1515=CARTESIAN_POINT ( 'NONE',  ( -34.88460058024264043, 16.28046363954882736, -1.493845543551999944 ) ) ;
#1516=DIRECTION ( 'NONE',  ( 0.9999836672264332815, -0.005715354789845002517, 0.000000000000000000 ) ) ;
#1517=CARTESIAN_POINT ( 'NONE',  ( 31.14423615379030608, -4.720863734206129259, 2.999999999999995559 ) ) ;
#1518=CARTESIAN_POINT ( 'NONE',  ( 43.45632180942044442, -94.90042465344848210, -3.001370543551634906 ) ) ;
#1520=CYLINDRICAL_SURFACE ( 'NONE', #3731, 6.300000000000000711 ) ;
#1521=ORIENTED_EDGE ( 'NONE', *, *, #4334, .T. ) ;
#1522=VERTEX_POINT ( 'NONE', #1199 ) ;
#1523=CARTESIAN_POINT ( 'NONE',  ( 1.714606436953501688E-17, 2.999951001679301835E-15, 0.000000000000000000 ) ) ;
#1524=DIRECTION ( 'NONE',  ( -4.026247463476719020E-15, 1.023028141612472829E-15, -1.000000000000000000 ) ) ;
#1526=LINE ( 'NONE', #7244, #1465 ) ;
#1528=ORIENTED_EDGE ( 'NONE', *, *, #6768, .F. ) ;
#1531=ORIENTED_EDGE ( 'NONE', *, *, #3695, .F. ) ;
#1537=ORIENTED_EDGE ( 'NONE', *, *, #76, .F. ) ;
#1540=EDGE_CURVE ( 'NONE', #6097, #901, #5947, .T. ) ;
#1541=ORIENTED_EDGE ( 'NONE', *, *, #2264, .F. ) ;
#1542=PLANE ( 'NONE',  #3149 ) ;
#1543=CARTESIAN_POINT ( 'NONE',  ( -17.21006346072928750, 13.86884027412869180, -2.230393353321906247 ) ) ;
#1545=CARTESIAN_POINT ( 'NONE',  ( 15.39542127499540136, -35.83857563806657964, 2.999999999999964473 ) ) ;
#1546=EDGE_CURVE ( 'NONE', #212, #6210, #1678, .T. ) ;
#1547=VERTEX_POINT ( 'NONE', #7359 ) ;
#1550=DIRECTION ( 'NONE',  ( 5.715354789845004342E-18, 9.999836672264337477E-16, -1.000000000000000000 ) ) ;
#1554=ORIENTED_EDGE ( 'NONE', *, *, #6544, .T. ) ;
#1556=DIRECTION ( 'NONE',  ( 0.02358931830619094214, -0.9997217333147505602, -9.995705837626804294E-16 ) ) ;
#1558=CARTESIAN_POINT ( 'NONE',  ( 7.529070345495034289, 16.11642554373085900, 3.000000000000015987 ) ) ;
#1564=EDGE_LOOP ( 'NONE', ( #7406, #1608, #3074, #586 ) ) ;
#1575=ORIENTED_EDGE ( 'NONE', *, *, #6853, .F. ) ;
#1576=CARTESIAN_POINT ( 'NONE',  ( 9.018117650298766108, 16.81805756487467107, -0.3999035282154979054 ) ) ;
#1577=CIRCLE ( 'NONE', #4104, 1.100000000000000755 ) ;
#1580=CARTESIAN_POINT ( 'NONE',  ( 11.65361085287446663, 10.55667343862480578, 1.040834085586084257E-14 ) ) ;
#1582=AXIS2_PLACEMENT_3D ( 'NONE', #2900, #6313, #5146 ) ;
#1583=ORIENTED_EDGE ( 'NONE', *, *, #5545, .F. ) ;
#1585=VECTOR ( 'NONE', #4910, 1000.000000000000227 ) ;
#1587=EDGE_CURVE ( 'NONE', #6014, #5486, #2985, .T. ) ;
#1588=CYLINDRICAL_SURFACE ( 'NONE', #5449, 3.750000000000000000 ) ;
#1589=EDGE_CURVE ( 'NONE', #6736, #2542, #6900, .T. ) ;
#1593=CARTESIAN_POINT ( 'NONE',  ( 14.63763862841553376, 20.11382921380832656, 0.006154456448485313980 ) ) ;
#1598=CARTESIAN_POINT ( 'NONE',  ( -13.25471347244850051, 13.28966623998220520, -0.1388209971588587888 ) ) ;
#1601=AXIS2_PLACEMENT_3D ( 'NONE', #5028, #3777, #7311 ) ;
#1603=VECTOR ( 'NONE', #1165, 1000.000000000000227 ) ;
#1608=ORIENTED_EDGE ( 'NONE', *, *, #6789, .T. ) ;
#1610=VECTOR ( 'NONE', #4576, 1000.000000000000114 ) ;
#1611=CYLINDRICAL_SURFACE ( 'NONE', #2192, 2.999999999999999556 ) ;
#1620=VECTOR ( 'NONE', #3144, 1000.000000000000000 ) ;
#1622=DIRECTION ( 'NONE',  ( -5.715354789845005112E-18, -9.999836672264339449E-16, 1.000000000000000000 ) ) ;
#1627=FACE_OUTER_BOUND ( 'NONE', #4793, .T. ) ;
#1630=ORIENTED_EDGE ( 'NONE', *, *, #935, .F. ) ;
#1633=CARTESIAN_POINT ( 'NONE',  ( -15.00216760413269945, 6.625337177075936168, 6.505213034913026604E-15 ) ) ;
#1635=CYLINDRICAL_SURFACE ( 'NONE', #5207, 6.299999999999998934 ) ;
#1642=ORIENTED_EDGE ( 'NONE', *, *, #4346, .T. ) ;
#1646=DIRECTION ( 'NONE',  ( 0.7411265327553895332, 0.6713653717953992350, 6.755902076156661002E-16 ) ) ;
#1647=DIRECTION ( 'NONE',  ( 0.7411265327553895332, 0.6713653717953992350, 6.755902076156661002E-16 ) ) ;
#1651=CARTESIAN_POINT ( 'NONE',  ( 12.99837876291259064, -32.41640519645540053, -3.252606517456513302E-14 ) ) ;
#1653=CARTESIAN_POINT ( 'NONE',  ( 13.75614703236065672, 19.53106228095526475, -2.928563623636441182 ) ) ;
#1654=DIRECTION ( 'NONE',  ( 0.6713653717953971256, -0.7411265327553914206, -7.372773368101209313E-16 ) ) ;
#1656=PLANE ( 'NONE',  #125 ) ;
#1660=ADVANCED_FACE ( 'NONE', ( #3667, #697 ), #670, .T. ) ;
#1663=FACE_OUTER_BOUND ( 'NONE', #1899, .T. ) ;
#1667=LINE ( 'NONE', #4621, #857 ) ;
#1668=DIRECTION ( 'NONE',  ( -0.4039838799357113319, -0.9147661038495518149, -9.170600743851232967E-16 ) ) ;
#1669=EDGE_CURVE ( 'NONE', #6942, #1547, #4737, .T. ) ;
#1676=ORIENTED_EDGE ( 'NONE', *, *, #2776, .T. ) ;
#1678=LINE ( 'NONE', #3976, #4246 ) ;
#1680=FACE_OUTER_BOUND ( 'NONE', #7138, .T. ) ;
#1683=CARTESIAN_POINT ( 'NONE',  ( 22.42915535073480982, 21.39736943723329432, -1.493845543551513444 ) ) ;
#1686=VERTEX_POINT ( 'NONE', #3094 ) ;
#1688=VERTEX_POINT ( 'NONE', #1277 ) ;
#1692=CIRCLE ( 'NONE', #5911, 0.7500000000000000000 ) ;
#1694=CARTESIAN_POINT ( 'NONE',  ( -13.76286933773225130, 13.32929763200878881, -0.3999035282155013471 ) ) ;
#1695=CARTESIAN_POINT ( 'NONE',  ( 13.14859132361180194, 19.41219719266456423, 0.4060579846640096635 ) ) ;
#1701=VECTOR ( 'NONE', #1069, 1000.000000000000000 ) ;
#1707=AXIS2_PLACEMENT_3D ( 'NONE', #4115, #1266, #3547 ) ;
#1708=ADVANCED_FACE ( 'NONE', ( #1340 ), #3555, .F. ) ;
#1714=FACE_OUTER_BOUND ( 'NONE', #6457, .T. ) ;
#1715=ORIENTED_EDGE ( 'NONE', *, *, #2768, .F. ) ;
#1718=EDGE_CURVE ( 'NONE', #5680, #3357, #5563, .T. ) ;
#1719=VECTOR ( 'NONE', #2428, 999.9999999999998863 ) ;
#1724=ORIENTED_EDGE ( 'NONE', *, *, #3118, .T. ) ;
#1725=FACE_OUTER_BOUND ( 'NONE', #2424, .T. ) ;
#1729=VECTOR ( 'NONE', #6046, 1000.000000000000227 ) ;
#1731=ORIENTED_EDGE ( 'NONE', *, *, #6011, .F. ) ;
#1732=ORIENTED_EDGE ( 'NONE', *, *, #5730, .T. ) ;
#1733=EDGE_CURVE ( 'NONE', #5350, #6877, #627, .T. ) ;
#1737=AXIS2_PLACEMENT_3D ( 'NONE', #5345, #3726, #2030 ) ;
#1738=FACE_OUTER_BOUND ( 'NONE', #6531, .T. ) ;
#1740=DIRECTION ( 'NONE',  ( -0.9879743132267128081, -0.1546180985661290141, -1.602621969470799848E-16 ) ) ;
#1741=EDGE_LOOP ( 'NONE', ( #2241, #2822, #2285, #6053 ) ) ;
#1745=CARTESIAN_POINT ( 'NONE',  ( -11.40395268922818062, 1.749910050107414738, 1.734723475976807094E-15 ) ) ;
#1749=LINE ( 'NONE', #4045, #1846 ) ;
#1754=LINE ( 'NONE', #4080, #1365 ) ;
#1759=ORIENTED_EDGE ( 'NONE', *, *, #5, .T. ) ;
#1760=ORIENTED_EDGE ( 'NONE', *, *, #1281, .F. ) ;
#1762=LINE ( 'NONE', #5760, #642 ) ;
#1763=CARTESIAN_POINT ( 'NONE',  ( 7.529070345495034289, 16.11642554373085900, 3.000000000000015987 ) ) ;
#1769=ORIENTED_EDGE ( 'NONE', *, *, #1400, .F. ) ;
#1770=CARTESIAN_POINT ( 'NONE',  ( 41.70778007397900211, -94.98992620957551480, -9.454242944073598665E-14 ) ) ;
#1771=DIRECTION ( 'NONE',  ( -0.4039838799357104437, -0.9147661038495520369, -1.600849619044994772E-16 ) ) ;
#1776=CARTESIAN_POINT ( 'NONE',  ( 26.67188031194815068, 24.16129507000589527, -2.993845543551515664 ) ) ;
#1777=ORIENTED_EDGE ( 'NONE', *, *, #1281, .T. ) ;
#1780=EDGE_CURVE ( 'NONE', #4731, #6736, #6713, .T. ) ;
#1787=DIRECTION ( 'NONE',  ( -0.8039121061460989814, 0.3550279469270786747, -0.4771587602596088495 ) ) ;
#1792=ORIENTED_EDGE ( 'NONE', *, *, #2970, .T. ) ;
#1795=CARTESIAN_POINT ( 'NONE',  ( 11.65361085287446663, 10.55667343862480223, 3.000000000000010658 ) ) ;
#1796=CARTESIAN_POINT ( 'NONE',  ( 28.12455780688322449, -37.01391159201033787, -3.686287386450715076E-14 ) ) ;
#1800=AXIS2_PLACEMENT_3D ( 'NONE', #4906, #1425, #6085 ) ;
#1801=EDGE_CURVE ( 'NONE', #553, #5128, #5448, .T. ) ;
#1804=CARTESIAN_POINT ( 'NONE',  ( 22.42915535073480982, 21.39736943723329432, -1.493845543551513444 ) ) ;
#1809=VECTOR ( 'NONE', #1622, 1000.000000000000000 ) ;
#1810=EDGE_CURVE ( 'NONE', #184, #5945, #3298, .T. ) ;
#1812=LINE ( 'NONE', #5254, #6845 ) ;
#1817=DIRECTION ( 'NONE',  ( 0.4039838799357100552, 0.9147661038495522590, 1.399039571475124858E-16 ) ) ;
#1819=EDGE_CURVE ( 'NONE', #1942, #3815, #6056, .T. ) ;
#1820=LINE ( 'NONE', #4760, #1253 ) ;
#1827=ORIENTED_EDGE ( 'NONE', *, *, #1427, .T. ) ;
#1828=DIRECTION ( 'NONE',  ( 0.7411265327553895332, 0.6713653717953992350, 6.755902076156662974E-16 ) ) ;
#1830=CARTESIAN_POINT ( 'NONE',  ( 7.529070345495034289, 16.11642554373086256, 1.604619215278546562E-14 ) ) ;
#1834=ORIENTED_EDGE ( 'NONE', *, *, #2768, .T. ) ;
#1836=PLANE ( 'NONE',  #40 ) ;
#1837=VECTOR ( 'NONE', #5194, 1000.000000000000114 ) ;
#1838=CARTESIAN_POINT ( 'NONE',  ( -11.40395268922818062, 1.749910050107411630, 3.000000000000001776 ) ) ;
#1846=VECTOR ( 'NONE', #6346, 1000.000000000000000 ) ;
#1852=DIRECTION ( 'NONE',  ( 0.2098925886716649092, 0.9716434517700405227, -0.1088765532752961201 ) ) ;
#1855=CARTESIAN_POINT ( 'NONE',  ( 39.32685927492619982, -94.35036853610694152, 2.999999999999905853 ) ) ;
#1857=CARTESIAN_POINT ( 'NONE',  ( -7.741417275248890562, 12.33509147838778830, 1.214306433183764966E-14 ) ) ;
#1858=CARTESIAN_POINT ( 'NONE',  ( 4.492111197601039052, 14.38610368760445546, 1.431146867680865853E-14 ) ) ;
#1867=CARTESIAN_POINT ( 'NONE',  ( -16.21021049057420882, 1.692961427013494724, -2.993845543551527655 ) ) ;
#1874=DIRECTION ( 'NONE',  ( -5.715354789845005112E-18, -9.999836672264339449E-16, 1.000000000000000000 ) ) ;
#1877=CARTESIAN_POINT ( 'NONE',  ( 15.94457129749017277, -41.07922723232461237, 2.999999999999958700 ) ) ;
#1880=DIRECTION ( 'NONE',  ( -5.715354789845005112E-18, -9.999836672264339449E-16, 1.000000000000000000 ) ) ;
#1882=ORIENTED_EDGE ( 'NONE', *, *, #491, .T. ) ;
#1884=ADVANCED_FACE ( 'NONE', ( #356 ), #2648, .T. ) ;
#1891=ORIENTED_EDGE ( 'NONE', *, *, #2536, .T. ) ;
#1898=ORIENTED_EDGE ( 'NONE', *, *, #3686, .F. ) ;
#1899=EDGE_LOOP ( 'NONE', ( #657, #4674, #251, #1937 ) ) ;
#1910=CARTESIAN_POINT ( 'NONE',  ( 14.63763862841555330, 20.11382921380837629, 0.006154456448490084469 ) ) ;
#1911=CARTESIAN_POINT ( 'NONE',  ( -16.40387102536037744, 1.778486824056639826, 1.734723475976807094E-15 ) ) ;
#1913=STYLED_ITEM ( 'NONE', ( #4650 ), #4713 ) ;
#1920=DIRECTION ( 'NONE',  ( -0.9999836672264335036, 0.005715354789845003385, 1.110223024625156047E-16 ) ) ;
#1928=EDGE_CURVE ( 'NONE', #4359, #427, #1667, .T. ) ;
#1930=VERTEX_POINT ( 'NONE', #548 ) ;
#1932=AXIS2_PLACEMENT_3D ( 'NONE', #5358, #2482, #3176 ) ;
#1934=DIRECTION ( 'NONE',  ( -5.715354789845005112E-18, -9.999836672264339449E-16, 1.000000000000000000 ) ) ;
#1935=DIRECTION ( 'NONE',  ( 0.4364886600403651840, -0.1927644473149899840, -0.8788171126619650497 ) ) ;
#1937=ORIENTED_EDGE ( 'NONE', *, *, #892, .T. ) ;
#1939=EDGE_CURVE ( 'NONE', #5128, #320, #5787, .T. ) ;
#1940=EDGE_CURVE ( 'NONE', #5032, #4548, #3322, .T. ) ;
#1942=VERTEX_POINT ( 'NONE', #6205 ) ;
#1944=CIRCLE ( 'NONE', #5579, 6.299999999999998934 ) ;
#1948=CARTESIAN_POINT ( 'NONE',  ( -34.88460058024262622, 16.28046363954885933, -2.243845543551999722 ) ) ;
#1950=VECTOR ( 'NONE', #3402, 1000.000000000000000 ) ;
#1951=EDGE_CURVE ( 'NONE', #7317, #3224, #3925, .T. ) ;
#1953=ORIENTED_EDGE ( 'NONE', *, *, #1587, .T. ) ;
#1955=CARTESIAN_POINT ( 'NONE',  ( 14.63763862841553376, 20.11382921380832656, 0.006154456448485313980 ) ) ;
#1962=DIRECTION ( 'NONE',  ( -1.046706025223848628E-16, 1.111638688234981601E-15, -1.000000000000000000 ) ) ;
#1965=ORIENTED_EDGE ( 'NONE', *, *, #5377, .F. ) ;
#1968=CARTESIAN_POINT ( 'NONE',  ( 43.95483829995806957, -94.87490738911687060, -9.454242944073598665E-14 ) ) ;
#1976=FACE_OUTER_BOUND ( 'NONE', #4311, .T. ) ;
#1977=EDGE_CURVE ( 'NONE', #3563, #3666, #4230, .T. ) ;
#1986=EDGE_CURVE ( 'NONE', #4548, #2317, #2565, .T. ) ;
#1987=PLANE ( 'NONE',  #3022 ) ;
#1992=VERTEX_POINT ( 'NONE', #5110 ) ;
#1993=DIRECTION ( 'NONE',  ( -0.9828140593167949968, 0.1845982795403122156, 4.010227384219995304E-16 ) ) ;
#1996=ADVANCED_FACE ( 'NONE', ( #7391 ), #1635, .T. ) ;
#1997=CARTESIAN_POINT ( 'NONE',  ( 39.48483786921892857, -95.33781693134928048, 2.999999999999904965 ) ) ;
#2000=FACE_OUTER_BOUND ( 'NONE', #4206, .T. ) ;
#2001=EDGE_LOOP ( 'NONE', ( #5157, #1521, #1295, #1537 ) ) ;
#2003=EDGE_LOOP ( 'NONE', ( #1531, #353, #666, #7297 ) ) ;
#2014=FACE_OUTER_BOUND ( 'NONE', #4851, .T. ) ;
#2020=VERTEX_POINT ( 'NONE', #1110 ) ;
#2025=CIRCLE ( 'NONE', #1090, 140.0000000000000000 ) ;
#2027=CARTESIAN_POINT ( 'NONE',  ( -7.741417275248890562, 12.33509147838778830, 1.214306433183764966E-14 ) ) ;
#2028=CARTESIAN_POINT ( 'NONE',  ( -12.11759654540111875, 13.15705282150456590, 3.000000000000012879 ) ) ;
#2030=DIRECTION ( 'NONE',  ( 5.715354789845005112E-18, 9.999836672264339449E-16, -1.000000000000000000 ) ) ;
#2031=AXIS2_PLACEMENT_3D ( 'NONE', #6933, #5812, #2481 ) ;
#2037=ORIENTED_EDGE ( 'NONE', *, *, #6968, .T. ) ;
#2038=ORIENTED_EDGE ( 'NONE', *, *, #175, .F. ) ;
#2039=AXIS2_PLACEMENT_3D ( 'NONE', #2672, #4489, #6704 ) ;
#2040=DIRECTION ( 'NONE',  ( -5.715354789845005112E-18, -9.999836672264339449E-16, 1.000000000000000000 ) ) ;
#2046=ORIENTED_EDGE ( 'NONE', *, *, #2737, .T. ) ;
#2049=FACE_OUTER_BOUND ( 'NONE', #2128, .T. ) ;
#2055=ORIENTED_EDGE ( 'NONE', *, *, #3915, .T. ) ;
#2062=CARTESIAN_POINT ( 'NONE',  ( 18.47982041150265431, -39.47532202006953383, -3.946495907847236140E-14 ) ) ;
#2067=AXIS2_PLACEMENT_3D ( 'NONE', #3794, #2629, #6116 ) ;
#2071=EDGE_CURVE ( 'NONE', #3496, #6686, #163, .T. ) ;
#2075=LINE ( 'NONE', #6125, #5574 ) ;
#2078=CIRCLE ( 'NONE', #6187, 2.249999999999996891 ) ;
#2079=ORIENTED_EDGE ( 'NONE', *, *, #5189, .F. ) ;
#2080=LINE ( 'NONE', #6129, #6508 ) ;
#2081=AXIS2_PLACEMENT_3D ( 'NONE', #6817, #3998, #3955 ) ;
#2084=VECTOR ( 'NONE', #3167, 1000.000000000000114 ) ;
#2089=FACE_OUTER_BOUND ( 'NONE', #7077, .T. ) ;
#2092=CIRCLE ( 'NONE', #3656, 11.50000000000000178 ) ;
#2098=LINE ( 'NONE', #6656, #3896 ) ;
#2101=FACE_OUTER_BOUND ( 'NONE', #3698, .T. ) ;
#2105=ORIENTED_EDGE ( 'NONE', *, *, #4355, .T. ) ;
#2106=CARTESIAN_POINT ( 'NONE',  ( 11.37011796090756555, -1.723489934710178861, 2.999999999999998224 ) ) ;
#2108=DIRECTION ( 'NONE',  ( -5.715354789845005112E-18, -9.999836672264339449E-16, 1.000000000000000000 ) ) ;
#2112=CARTESIAN_POINT ( 'NONE',  ( 15.39542127499540136, -35.83857563806657964, -3.556183125752454544E-14 ) ) ;
#2115=CARTESIAN_POINT ( 'NONE',  ( 41.70778007397900211, -94.98992620957551480, 2.999999999999905409 ) ) ;
#2117=DIRECTION ( 'NONE',  ( -5.715354789845005112E-18, -9.999836672264339449E-16, 1.000000000000000000 ) ) ;
#2119=ORIENTED_EDGE ( 'NONE', *, *, #6156, .T. ) ;
#2127=ORIENTED_EDGE ( 'NONE', *, *, #310, .T. ) ;
#2128=EDGE_LOOP ( 'NONE', ( #6898, #105, #4222, #7186 ) ) ;
#2144=VECTOR ( 'NONE', #5924, 1000.000000000000227 ) ;
#2146=FACE_OUTER_BOUND ( 'NONE', #6290, .T. ) ;
#2151=LINE ( 'NONE', #6099, #5825 ) ;
#2158=ORIENTED_EDGE ( 'NONE', *, *, #15, .T. ) ;
#2159=EDGE_LOOP ( 'NONE', ( #4458, #6760, #2983, #5912 ) ) ;
#2160=CARTESIAN_POINT ( 'NONE',  ( -18.11931019897951955, 14.08535735325398619, -2.729487737349305831 ) ) ;
#2161=ORIENTED_EDGE ( 'NONE', *, *, #206, .F. ) ;
#2165=DIRECTION ( 'NONE',  ( -5.715354789845005112E-18, -9.999836672264339449E-16, 1.000000000000000000 ) ) ;
#2172=EDGE_CURVE ( 'NONE', #5715, #1377, #2786, .T. ) ;
#2174=CIRCLE ( 'NONE', #6399, 20.00000000000000000 ) ;
#2179=DIRECTION ( 'NONE',  ( 0.4364886600403651840, -0.1927644473149899840, -0.8788171126619650497 ) ) ;
#2183=FACE_OUTER_BOUND ( 'NONE', #250, .T. ) ;
#2187=CIRCLE ( 'NONE', #4239, 147.0000000000000000 ) ;
#2188=CARTESIAN_POINT ( 'NONE',  ( -13.76286933773225130, 13.32929763200878881, -0.3999035282155013471 ) ) ;
#2190=CARTESIAN_POINT ( 'NONE',  ( 25.15036705625666258, 26.15624279088187265, 2.645453300864630819E-14 ) ) ;
#2192=AXIS2_PLACEMENT_3D ( 'NONE', #5539, #6611, #4470 ) ;
#2193=LINE ( 'NONE', #2867, #1950 ) ;
#2196=AXIS2_PLACEMENT_3D ( 'NONE', #2934, #679, #1176 ) ;
#2199=ORIENTED_EDGE ( 'NONE', *, *, #5966, .T. ) ;
#2204=VERTEX_POINT ( 'NONE', #1148 ) ;
#2208=FACE_OUTER_BOUND ( 'NONE', #4439, .T. ) ;
#2211=ORIENTED_EDGE ( 'NONE', *, *, #5854, .F. ) ;
#2215=EDGE_CURVE ( 'NONE', #6877, #6097, #2260, .T. ) ;
#2222=ORIENTED_EDGE ( 'NONE', *, *, #5148, .F. ) ;
#2223=ORIENTED_EDGE ( 'NONE', *, *, #3784, .F. ) ;
#2225=EDGE_CURVE ( 'NONE', #6135, #321, #5322, .T. ) ;
#2227=CARTESIAN_POINT ( 'NONE',  ( 39.32685927492619982, -94.35036853610694152, -9.410874857174178487E-14 ) ) ;
#2236=DIRECTION ( 'NONE',  ( -1.850371707708594129E-14, -4.394632805807911095E-14, 1.000000000000000000 ) ) ;
#2241=ORIENTED_EDGE ( 'NONE', *, *, #6655, .F. ) ;
#2245=DIRECTION ( 'NONE',  ( 0.9147661038495522590, -0.4039838799357101107, 0.000000000000000000 ) ) ;
#2253=CARTESIAN_POINT ( 'NONE',  ( -20.83603634162975737, 9.201721367189403367, 0.4060579846639940094 ) ) ;
#2254=CARTESIAN_POINT ( 'NONE',  ( 18.47982041150265431, -39.47532202006953383, 2.999999999999960476 ) ) ;
#2258=LINE ( 'NONE', #4605, #6391 ) ;
#2260=LINE ( 'NONE', #1745, #5571 ) ;
#2264=EDGE_CURVE ( 'NONE', #2912, #6662, #269, .T. ) ;
#2266=ORIENTED_EDGE ( 'NONE', *, *, #4302, .F. ) ;
#2274=ADVANCED_FACE ( 'NONE', ( #605 ), #1588, .F. ) ;
#2281=DIRECTION ( 'NONE',  ( -5.715354789845005112E-18, -9.999836672264339449E-16, 1.000000000000000000 ) ) ;
#2285=ORIENTED_EDGE ( 'NONE', *, *, #3915, .F. ) ;
#2289=DIRECTION ( 'NONE',  ( -5.715354789845005112E-18, -9.999836672264339449E-16, 1.000000000000000000 ) ) ;
#2290=LINE ( 'NONE', #6334, #4749 ) ;
#2291=CARTESIAN_POINT ( 'NONE',  ( -16.40387102536037744, 1.778486824056639826, 1.734723475976807094E-15 ) ) ;
#2294=ORIENTED_EDGE ( 'NONE', *, *, #3052, .F. ) ;
#2295=DIRECTION ( 'NONE',  ( -5.715354789845005112E-18, -9.999836672264339449E-16, 1.000000000000000000 ) ) ;
#2301=VECTOR ( 'NONE', #1556, 1000.000000000000114 ) ;
#2307=DIRECTION ( 'NONE',  ( 0.1546180985661289864, -0.9879743132267128081, -9.870744795757291736E-16 ) ) ;
#2310=AXIS2_PLACEMENT_3D ( 'NONE', #924, #3737, #6684 ) ;
#2311=DIRECTION ( 'NONE',  ( -0.8545275983175482093, -0.5194059912184716410, -5.242814362801270410E-16 ) ) ;
#2314=B_SPLINE_CURVE_WITH_KNOTS ( 'NONE', 3,
 ( #1543, #5624, #457, #376 ),
 .UNSPECIFIED., .F., .F.,
 ( 4, 4 ),
 ( 0.000000000000000000, 1.000000000000000000 ),
 .UNSPECIFIED. ) ;
#2317=VERTEX_POINT ( 'NONE', #1218 ) ;
#2318=VERTEX_POINT ( 'NONE', #3046 ) ;
#2319=VECTOR ( 'NONE', #5639, 1000.000000000000000 ) ;
#2324=CARTESIAN_POINT ( 'NONE',  ( 24.99346688245966419, 26.01411140189437532, -2.993845543551503674 ) ) ;
#2336=FACE_OUTER_BOUND ( 'NONE', #1233, .T. ) ;
#2339=CYLINDRICAL_SURFACE ( 'NONE', #5950, 5.000000000000000000 ) ;
#2340=DIRECTION ( 'NONE',  ( 0.9999836672264332815, -0.005715354789845002517, 0.000000000000000000 ) ) ;
#2341=CARTESIAN_POINT ( 'NONE',  ( 12.15447797363371052, 11.01039466689934443, 1.127570259384924611E-14 ) ) ;
#2344=AXIS2_PLACEMENT_3D ( 'NONE', #187, #5308, #641 ) ;
#2345=ADVANCED_FACE ( 'NONE', ( #5923 ), #2485, .T. ) ;
#2347=PLANE ( 'NONE',  #2081 ) ;
#2349=CARTESIAN_POINT ( 'NONE',  ( -7.922926035662746003, 12.41525034409755612, 2.701156757981117984 ) ) ;
#2350=ORIENTED_EDGE ( 'NONE', *, *, #6966, .F. ) ;
#2352=CARTESIAN_POINT ( 'NONE',  ( 7.529070345495034289, 16.11642554373085900, 3.000000000000015987 ) ) ;
#2361=CARTESIAN_POINT ( 'NONE',  ( 15.82006518139326978, 14.33094549030128029, -2.230393353321955541 ) ) ;
#2366=ORIENTED_EDGE ( 'NONE', *, *, #3653, .T. ) ;
#2367=DIRECTION ( 'NONE',  ( -0.4039838799357098331, -0.9147661038495523700, -8.673617379884154787E-16 ) ) ;
#2369=DIRECTION ( 'NONE',  ( 0.9999836672264332815, -0.005715354789845002517, 0.000000000000000000 ) ) ;
#2373=ORIENTED_EDGE ( 'NONE', *, *, #621, .T. ) ;
#2374=EDGE_CURVE ( 'NONE', #5998, #1992, #2669, .T. ) ;
#2375=ADVANCED_FACE ( 'NONE', ( #4789 ), #3006, .T. ) ;
#2378=DIRECTION ( 'NONE',  ( 5.715354789845005112E-18, 9.999836672264339449E-16, -1.000000000000000000 ) ) ;
#2381=DIRECTION ( 'NONE',  ( 0.9999836672264332815, -0.005715354789845002517, 0.000000000000000000 ) ) ;
#2387=ORIENTED_EDGE ( 'NONE', *, *, #749, .F. ) ;
#2398=EDGE_CURVE ( 'NONE', #4056, #5232, #4136, .T. ) ;
#2399=FACE_OUTER_BOUND ( 'NONE', #4848, .T. ) ;
#2401=DIRECTION ( 'NONE',  ( -0.9999836672264333925, 0.005715354789844388425, 0.000000000000000000 ) ) ;
#2407=CARTESIAN_POINT ( 'NONE',  ( 0.000000000000000000, 0.000000000000000000, 3.000000000000000000 ) ) ;
#2412=ORIENTED_EDGE ( 'NONE', *, *, #7033, .T. ) ;
#2424=EDGE_LOOP ( 'NONE', ( #6067, #4558 ) ) ;
#2428=DIRECTION ( 'NONE',  ( 0.4039838799357093335, 0.9147661038495527031, 1.550530988647994607E-16 ) ) ;
#2430=CARTESIAN_POINT ( 'NONE',  ( 13.32147353159843028, 12.06754263290683937, -0.3999035282155026794 ) ) ;
#2431=VERTEX_POINT ( 'NONE', #3682 ) ;
#2434=( LENGTH_UNIT ( ) NAMED_UNIT ( * ) SI_UNIT ( .MILLI., .METRE. ) );
#2436=CIRCLE ( 'NONE', #7007, 17.99999999999999645 ) ;
#2438=CIRCLE ( 'NONE', #277, 2.999999999999999556 ) ;
#2441=PRODUCT_DEFINITION_FORMATION_WITH_SPECIFIED_SOURCE ( 'ANY', '', #196, .NOT_KNOWN. ) ;
#2443=ORIENTED_EDGE ( 'NONE', *, *, #6156, .F. ) ;
#2444=EDGE_CURVE ( 'NONE', #4550, #106, #4844, .T. ) ;
#2449=DIRECTION ( 'NONE',  ( 0.4039838799357101107, 0.9147661038495522590, 4.900000000000001209E-14 ) ) ;
#2453=ORIENTED_EDGE ( 'NONE', *, *, #5246, .F. ) ;
#2468=ORIENTED_EDGE ( 'NONE', *, *, #4815, .F. ) ;
#2473=LINE ( 'NONE', #733, #2084 ) ;
#2478=CARTESIAN_POINT ( 'NONE',  ( -22.27644891976294161, 9.837844043328900057, 3.306154456448478829 ) ) ;
#2479=CARTESIAN_POINT ( 'NONE',  ( 8.411763394295572738, 16.69999280642484507, 3.000000000000017764 ) ) ;
#2481=DIRECTION ( 'NONE',  ( -0.9999836672264332815, 0.005715354789845002517, 0.000000000000000000 ) ) ;
#2482=DIRECTION ( 'NONE',  ( -5.715354789845005112E-18, -9.999836672264339449E-16, 1.000000000000000000 ) ) ;
#2485=PLANE ( 'NONE',  #3264 ) ;
#2486=CARTESIAN_POINT ( 'NONE',  ( 24.99346688245966419, 26.01411140189437177, 0.006154456448490951831 ) ) ;
#2493=ADVANCED_FACE ( 'NONE', ( #7150 ), #1987, .F. ) ;
#2498=ORIENTED_EDGE ( 'NONE', *, *, #3695, .T. ) ;
#2499=B_SPLINE_CURVE_WITH_KNOTS ( 'NONE', 3,
 ( #3937, #6284, #6876, #521 ),
 .UNSPECIFIED., .F., .F.,
 ( 4, 4 ),
 ( 0.000000000000000000, 1.000000000000000000 ),
 .UNSPECIFIED. ) ;
#2501=ORIENTED_EDGE ( 'NONE', *, *, #4079, .T. ) ;
#2506=ORIENTED_EDGE ( 'NONE', *, *, #3456, .F. ) ;
#2507=EDGE_LOOP ( 'NONE', ( #810, #2686, #1731, #5231 ) ) ;
#2508=EDGE_LOOP ( 'NONE', ( #6079, #3187, #2962, #2387 ) ) ;
#2509=ORIENTED_EDGE ( 'NONE', *, *, #5359, .F. ) ;
#2510=CARTESIAN_POINT ( 'NONE',  ( -28.32684271132307074, 12.56450996214350191, -1.493845543551522992 ) ) ;
#2516=AXIS2_PLACEMENT_3D ( 'NONE', #4827, #2378, #230 ) ;
#2517=ORIENTED_EDGE ( 'NONE', *, *, #5847, .T. ) ;
#2522=LINE ( 'NONE', #3609, #2144 ) ;
#2524=VECTOR ( 'NONE', #6152, 1000.000000000000114 ) ;
#2525=ORIENTED_EDGE ( 'NONE', *, *, #536, .T. ) ;
#2528=CARTESIAN_POINT ( 'NONE',  ( 22.93267937958154690, 20.84152453766645507, -1.493845543551514332 ) ) ;
#2536=EDGE_CURVE ( 'NONE', #6689, #138, #993, .T. ) ;
#2542=VERTEX_POINT ( 'NONE', #1796 ) ;
#2545=ADVANCED_FACE ( 'NONE', ( #1085 ), #4024, .F. ) ;
#2546=EDGE_CURVE ( 'NONE', #7283, #1547, #3978, .T. ) ;
#2548=FACE_OUTER_BOUND ( 'NONE', #1741, .T. ) ;
#2555=AXIS2_PLACEMENT_3D ( 'NONE', #2668, #4975, #6333 ) ;
#2556=EDGE_CURVE ( 'NONE', #1441, #6014, #2436, .T. ) ;
#2561=DIRECTION ( 'NONE',  ( 5.715354789845005112E-18, 9.999836672264339449E-16, -1.000000000000000000 ) ) ;
#2562=DIRECTION ( 'NONE',  ( 0.9999836672264332815, -0.005715354789845002517, 0.000000000000000000 ) ) ;
#2565=CIRCLE ( 'NONE', #6750, 0.7500000000000000000 ) ;
#2566=ORIENTED_EDGE ( 'NONE', *, *, #1733, .F. ) ;
#2568=DIRECTION ( 'NONE',  ( 5.715354789845005112E-18, 9.999836672264339449E-16, -1.000000000000000000 ) ) ;
#2569=AXIS2_PLACEMENT_3D ( 'NONE', #1683, #1646, #7363 ) ;
#2579=AXIS2_PLACEMENT_3D ( 'NONE', #6612, #6074, #5540 ) ;
#2581=DIRECTION ( 'NONE',  ( 5.715354789845005112E-18, 9.999836672264339449E-16, -1.000000000000000000 ) ) ;
#2583=ADVANCED_FACE ( 'NONE', ( #1680 ), #5271, .F. ) ;
#2589=DIRECTION ( 'NONE',  ( -0.5144810339903909124, 0.8512598437243096283, -0.1032760578577736621 ) ) ;
#2591=CARTESIAN_POINT ( 'NONE',  ( 19.34585819626726533, -40.86123582061801329, 2.999999999999959144 ) ) ;
#2595=ORIENTED_EDGE ( 'NONE', *, *, #161, .F. ) ;
#2597=ADVANCED_FACE ( 'NONE', ( #1725 ), #101, .T. ) ;
#2598=EDGE_CURVE ( 'NONE', #7172, #7317, #6818, .T. ) ;
#2600=EDGE_LOOP ( 'NONE', ( #98, #3783 ) ) ;
#2607=FACE_BOUND ( 'NONE', #4450, .T. ) ;
#2609=DIRECTION ( 'NONE',  ( -6.548793834854970868E-18, -1.145805836327743954E-15, -1.000000000000000000 ) ) ;
#2611=VERTEX_POINT ( 'NONE', #5161 ) ;
#2612=EDGE_LOOP ( 'NONE', ( #2105, #1042, #1732, #831 ) ) ;
#2613=CARTESIAN_POINT ( 'NONE',  ( -13.76286933773225130, 13.32929763200878881, -0.3999035282155013471 ) ) ;
#2614=CARTESIAN_POINT ( 'NONE',  ( 10.07902270299396008, 17.77910117033601978, 2.236547809770395911 ) ) ;
#2619=ORIENTED_EDGE ( 'NONE', *, *, #7361, .F. ) ;
#2621=ORIENTED_EDGE ( 'NONE', *, *, #6248, .T. ) ;
#2623=DIRECTION ( 'NONE',  ( -5.715354789845005112E-18, -9.999836672264339449E-16, 1.000000000000000000 ) ) ;
#2624=CARTESIAN_POINT ( 'NONE',  ( -22.85595574130830698, 4.627890847941666053, 0.4060579846639992274 ) ) ;
#2629=DIRECTION ( 'NONE',  ( -5.715354789845005112E-18, -9.999836672264339449E-16, 1.000000000000000000 ) ) ;
#2633=CARTESIAN_POINT ( 'NONE',  ( 12.99837876291259064, -32.41640519645540053, -3.252606517456513302E-14 ) ) ;
#2636=EDGE_CURVE ( 'NONE', #5945, #4029, #3450, .T. ) ;
#2638=CYLINDRICAL_SURFACE ( 'NONE', #4386, 0.7499999999999997780 ) ;
#2639=DIRECTION ( 'NONE',  ( 0.6713653717953970146, -0.7411265327553913096, -7.372773368101209313E-16 ) ) ;
#2640=CARTESIAN_POINT ( 'NONE',  ( -25.53008038988497930, -12.83396994533167756, -1.301042606982605321E-14 ) ) ;
#2641=CARTESIAN_POINT ( 'NONE',  ( -16.40387102536037744, 1.778486824056636939, 3.000000000000001776 ) ) ;
#2643=CARTESIAN_POINT ( 'NONE',  ( -14.38395162568180652, 6.352317343304404673, 6.071532165918824830E-15 ) ) ;
#2644=EDGE_LOOP ( 'NONE', ( #5023, #5527 ) ) ;
#2645=CARTESIAN_POINT ( 'NONE',  ( -19.02833027023232404, 14.48681530925147776, 0.1446440811472397281 ) ) ;
#2646=EDGE_CURVE ( 'NONE', #2710, #75, #26, .T. ) ;
#2648=CYLINDRICAL_SURFACE ( 'NONE', #6186, 11.50000000000000178 ) ;
#2649=CARTESIAN_POINT ( 'NONE',  ( 21.92563132188844932, 21.95321433679954026, -1.493845543551513444 ) ) ;
#2653=ORIENTED_EDGE ( 'NONE', *, *, #4815, .T. ) ;
#2656=ORIENTED_EDGE ( 'NONE', *, *, #2546, .F. ) ;
#2657=ORIENTED_EDGE ( 'NONE', *, *, #1351, .T. ) ;
#2658=ORIENTED_EDGE ( 'NONE', *, *, #6680, .F. ) ;
#2660=CARTESIAN_POINT ( 'NONE',  ( -19.13960539129976368, 14.35165484499600375, -2.993845543551525878 ) ) ;
#2667=PLANE ( 'NONE',  #34 ) ;
#2668=CARTESIAN_POINT ( 'NONE',  ( 24.80820526761568345, 22.47304504285837368, -8.815182418718737978 ) ) ;
#2669=CIRCLE ( 'NONE', #6633, 0.7499999999999872324 ) ;
#2672=CARTESIAN_POINT ( 'NONE',  ( 18.04796579205319063, 16.34913706177017190, 3.306154456448483714 ) ) ;
#2673=AXIS2_PLACEMENT_3D ( 'NONE', #2946, #6509, #3473 ) ;
#2674=EDGE_CURVE ( 'NONE', #4811, #5242, #4058, .T. ) ;
#2677=CARTESIAN_POINT ( 'NONE',  ( 11.65361085287446663, 10.55667343862480578, 1.040834085586084257E-14 ) ) ;
#2683=EDGE_CURVE ( 'NONE', #7093, #3534, #5218, .T. ) ;
#2686=ORIENTED_EDGE ( 'NONE', *, *, #609, .F. ) ;
#2687=FACE_OUTER_BOUND ( 'NONE', #891, .T. ) ;
#2688=AXIS2_PLACEMENT_3D ( 'NONE', #5173, #2179, #541 ) ;
#2696=PLANE ( 'NONE',  #4823 ) ;
#2697=EDGE_CURVE ( 'NONE', #7434, #3587, #1944, .T. ) ;
#2701=EDGE_LOOP ( 'NONE', ( #2266, #5296, #5800, #6705 ) ) ;
#2704=CARTESIAN_POINT ( 'NONE',  ( -17.66408190574286508, 13.97695476434122952, -2.479608496603234791 ) ) ;
#2705=CARTESIAN_POINT ( 'NONE',  ( 22.42915535073499811, 21.39736943723299945, -1.493845543551999944 ) ) ;
#2710=VERTEX_POINT ( 'NONE', #1411 ) ;
#2711=CARTESIAN_POINT ( 'NONE',  ( 3.603225912324908187, 20.45020204625077298, -3.299999999999978950 ) ) ;
#2715=LINE ( 'NONE', #2640, #2998 ) ;
#2717=CARTESIAN_POINT ( 'NONE',  ( 14.63763862841553376, 20.11382921380832656, -0.9938455435515094472 ) ) ;
#2718=EDGE_LOOP ( 'NONE', ( #7164, #1311, #5601, #2412 ) ) ;
#2723=DIRECTION ( 'NONE',  ( -0.02358931830619094214, 0.9997217333147506713, 9.995705837626806266E-16 ) ) ;
#2725=CYLINDRICAL_SURFACE ( 'NONE', #3260, 2.249999999999996891 ) ;
#2726=DIRECTION ( 'NONE',  ( -5.715354789845005112E-18, -9.999836672264339449E-16, 1.000000000000000000 ) ) ;
#2731=CARTESIAN_POINT ( 'NONE',  ( -20.16480223318149356, 14.61937842657788167, 0.006154456448484012937 ) ) ;
#2737=EDGE_CURVE ( 'NONE', #7172, #1441, #3095, .T. ) ;
#2747=ORIENTED_EDGE ( 'NONE', *, *, #4402, .F. ) ;
#2757=ADVANCED_FACE ( 'NONE', ( #5874 ), #178, .T. ) ;
#2758=ORIENTED_EDGE ( 'NONE', *, *, #1053, .T. ) ;
#2761=DIRECTION ( 'NONE',  ( -5.715354789845005112E-18, -9.999836672264339449E-16, 1.000000000000000000 ) ) ;
#2764=AXIS2_PLACEMENT_3D ( 'NONE', #3930, #4014, #4466 ) ;
#2765=CARTESIAN_POINT ( 'NONE',  ( -32.92087242456759100, 14.53869105662955796, -2.993845543551514776 ) ) ;
#2768=EDGE_CURVE ( 'NONE', #3946, #4056, #4237, .T. ) ;
#2769=EDGE_CURVE ( 'NONE', #1506, #3480, #5382, .T. ) ;
#2773=DIRECTION ( 'NONE',  ( -5.715354789845005112E-18, -9.999836672264339449E-16, 1.000000000000000000 ) ) ;
#2774=DIRECTION ( 'NONE',  ( -5.715354789845005112E-18, -9.999836672264339449E-16, 1.000000000000000000 ) ) ;
#2776=EDGE_CURVE ( 'NONE', #1000, #3480, #5409, .T. ) ;
#2778=ORIENTED_EDGE ( 'NONE', *, *, #3118, .F. ) ;
#2781=DIRECTION ( 'NONE',  ( 0.9999836672264335036, -0.005715354789845041548, 0.000000000000000000 ) ) ;
#2782=CARTESIAN_POINT ( 'NONE',  ( -18.51952944085035924, 14.44713361607365876, 0.4060579846639944535 ) ) ;
#2786=CIRCLE ( 'NONE', #4486, 0.7500000000000003331 ) ;
#2789=( GEOMETRIC_REPRESENTATION_CONTEXT ( 3 ) GLOBAL_UNCERTAINTY_ASSIGNED_CONTEXT ( ( #3056 ) ) GLOBAL_UNIT_ASSIGNED_CONTEXT ( ( #2434, #1347, #4096 ) ) REPRESENTATION_CONTEXT ( 'NONE', 'WORKASPACE' ) );
#2790=ORIENTED_EDGE ( 'NONE', *, *, #4686, .T. ) ;
#2792=CARTESIAN_POINT ( 'NONE',  ( -32.59768532061907109, 15.27050393970921327, -1.493845543551520327 ) ) ;
#2795=LINE ( 'NONE', #7393, #5338 ) ;
#2800=VECTOR ( 'NONE', #5789, 1000.000000000000227 ) ;
#2801=ORIENTED_EDGE ( 'NONE', *, *, #3234, .F. ) ;
#2805=ORIENTED_EDGE ( 'NONE', *, *, #2990, .F. ) ;
#2806=ADVANCED_FACE ( 'NONE', ( #6493 ), #6065, .F. ) ;
#2807=DIRECTION ( 'NONE',  ( -0.9999836672264333925, 0.005715354789844960016, 0.000000000000000000 ) ) ;
#2814=CARTESIAN_POINT ( 'NONE',  ( 7.529070345495034289, 16.11642554373086256, 1.604619215278546562E-14 ) ) ;
#2816=CARTESIAN_POINT ( 'NONE',  ( -19.52657036150863235, 8.623428025244454176, -2.230393353321931560 ) ) ;
#2819=DIRECTION ( 'NONE',  ( 0.5194059912184716410, -0.8545275983175482093, -8.515450519919942904E-16 ) ) ;
#2821=EDGE_LOOP ( 'NONE', ( #804, #5120, #2778, #518 ) ) ;
#2822=ORIENTED_EDGE ( 'NONE', *, *, #1819, .F. ) ;
#2829=DIRECTION ( 'NONE',  ( 6.276044648701490311E-18, 1.098084436444154719E-15, -1.000000000000000000 ) ) ;
#2833=CARTESIAN_POINT ( 'NONE',  ( 27.98760434640042050, 26.43260972569849443, -1.493845543551990174 ) ) ;
#2835=DIRECTION ( 'NONE',  ( -5.715354789845005112E-18, -9.999836672264339449E-16, 1.000000000000000000 ) ) ;
#2837=ORIENTED_EDGE ( 'NONE', *, *, #7104, .T. ) ;
#2844=LINE ( 'NONE', #5162, #287 ) ;
#2845=CARTESIAN_POINT ( 'NONE',  ( -7.672523287152989369, -8.566351989504937592, -8.673617379884035472E-15 ) ) ;
#2848=CARTESIAN_POINT ( 'NONE',  ( 8.041936255418978163, 16.36526498932675366, 2.068895131770362987E-14 ) ) ;
#2850=DIRECTION ( 'NONE',  ( -5.715354789845005112E-18, -9.999836672264339449E-16, 1.000000000000000000 ) ) ;
#2851=DIRECTION ( 'NONE',  ( 0.9999836672264332815, -0.005715354789845002517, 0.000000000000000000 ) ) ;
#2854=ORIENTED_EDGE ( 'NONE', *, *, #4440, .F. ) ;
#2859=DIRECTION ( 'NONE',  ( 0.9999836672264332815, -0.005715354789845002517, 0.000000000000000000 ) ) ;
#2861=DIRECTION ( 'NONE',  ( 5.715354789845005112E-18, 9.999836672264339449E-16, -1.000000000000000000 ) ) ;
#2863=EDGE_CURVE ( 'NONE', #89, #5783, #956, .T. ) ;
#2864=ADVANCED_FACE ( 'NONE', ( #6714 ), #3247, .T. ) ;
#2867=CARTESIAN_POINT ( 'NONE',  ( 39.32685927492619982, -94.35036853610694152, -9.410874857174178487E-14 ) ) ;
#2870=CARTESIAN_POINT ( 'NONE',  ( 12.68569177933871828, -46.07971015455952113, -4.597017211338538800E-14 ) ) ;
#2872=ORIENTED_EDGE ( 'NONE', *, *, #4593, .T. ) ;
#2874=EDGE_LOOP ( 'NONE', ( #1965, #6617, #4076, #4516 ) ) ;
#2878=DIRECTION ( 'NONE',  ( 0.9999836672264332815, -0.005715354789844959149, 0.000000000000000000 ) ) ;
#2880=PLANE ( 'NONE',  #4140 ) ;
#2888=DIRECTION ( 'NONE',  ( 0.9999836672264332815, -0.005715354789845002517, 0.000000000000000000 ) ) ;
#2890=ORIENTED_EDGE ( 'NONE', *, *, #1071, .T. ) ;
#2892=VECTOR ( 'NONE', #5670, 1000.000000000000000 ) ;
#2893=CARTESIAN_POINT ( 'NONE',  ( 11.37011796090756555, -1.723489934710175753, -1.734723475976807094E-15 ) ) ;
#2894=EDGE_CURVE ( 'NONE', #3657, #4478, #3174, .T. ) ;
#2900=CARTESIAN_POINT ( 'NONE',  ( -28.02385480137100160, 13.25058454003099939, -1.493845543551999944 ) ) ;
#2909=DIRECTION ( 'NONE',  ( -0.4039838799357104437, -0.9147661038495520369, -1.600849619044994772E-16 ) ) ;
#2912=VERTEX_POINT ( 'NONE', #5564 ) ;
#2917=DIRECTION ( 'NONE',  ( -0.005715354789845003385, -0.9999836672264335036, -2.228438827623913869E-16 ) ) ;
#2918=ADVANCED_FACE ( 'NONE', ( #358 ), #4394, .F. ) ;
#2924=AXIS2_PLACEMENT_3D ( 'NONE', #5873, #1828, #4130 ) ;
#2927=VERTEX_POINT ( 'NONE', #2649 ) ;
#2929=CARTESIAN_POINT ( 'NONE',  ( 14.29543924104632779, -35.83228874779774742, -3.556183125752454544E-14 ) ) ;
#2930=EDGE_CURVE ( 'NONE', #106, #6689, #4956, .T. ) ;
#2931=CARTESIAN_POINT ( 'NONE',  ( 7.529070345495034289, 16.11642554373085900, 3.000000000000015987 ) ) ;
#2934=CARTESIAN_POINT ( 'NONE',  ( 27.98760434640042050, 26.43260972569849443, -1.493845543551990174 ) ) ;
#2946=CARTESIAN_POINT ( 'NONE',  ( -16.56077119915742202, 1.636355435069145381, 0.006154456448471436192 ) ) ;
#2953=ORIENTED_EDGE ( 'NONE', *, *, #1499, .T. ) ;
#2957=DIRECTION ( 'NONE',  ( 0.6513146796332659472, 0.5900073775824578037, -0.4771587602596093491 ) ) ;
#2958=CARTESIAN_POINT ( 'NONE',  ( 7.529070345495034289, 16.11642554373085900, 2.000000000000016431 ) ) ;
#2961=ORIENTED_EDGE ( 'NONE', *, *, #1304, .T. ) ;
#2962=ORIENTED_EDGE ( 'NONE', *, *, #6294, .F. ) ;
#2963=EDGE_CURVE ( 'NONE', #6869, #3480, #3872, .T. ) ;
#2964=ADVANCED_FACE ( 'NONE', ( #323 ), #1397, .F. ) ;
#2966=DIRECTION ( 'NONE',  ( -0.9147661038495521479, 0.4039838799357104993, 3.987490689252507167E-16 ) ) ;
#2970=EDGE_CURVE ( 'NONE', #3589, #3446, #4850, .T. ) ;
#2972=CARTESIAN_POINT ( 'NONE',  ( 13.61290835672744848, 19.61678186576282812, 0.1446417891851695114 ) ) ;
#2976=ORIENTED_EDGE ( 'NONE', *, *, #7104, .F. ) ;
#2983=ORIENTED_EDGE ( 'NONE', *, *, #119, .F. ) ;
#2985=LINE ( 'NONE', #4279, #7008 ) ;
#2990=EDGE_CURVE ( 'NONE', #4056, #2431, #2151, .T. ) ;
#2991=VERTEX_POINT ( 'NONE', #4463 ) ;
#2998=VECTOR ( 'NONE', #4419, 1000.000000000000114 ) ;
#3000=CARTESIAN_POINT ( 'NONE',  ( -18.14656847176053844, 14.09764149780733966, -2.671436925771696114 ) ) ;
#3002=ADVANCED_FACE ( 'NONE', ( #6350 ), #1073, .F. ) ;
#3003=EDGE_CURVE ( 'NONE', #5506, #1000, #2795, .T. ) ;
#3005=VECTOR ( 'NONE', #5774, 999.9999999999998863 ) ;
#3006=B_SPLINE_SURFACE_WITH_KNOTS ( 'NONE', 1, 3, ( 
 ( #4753, #3543, #5361, #5286 ),
 ( #3608, #2972, #7073, #1910 ) ),
 .UNSPECIFIED., .F., .F., .F.,
 ( 2, 2 ),
 ( 4, 4 ),
 ( 0.000000000000000000, 1.000000000000000000 ),
 ( 0.000000000000000000, 1.000000000000000000 ),
 .UNSPECIFIED. ) ;
#3013=DIRECTION ( 'NONE',  ( 0.8545275983175482093, 0.5194059912184716410, 5.242814362801270410E-16 ) ) ;
#3020=ORIENTED_EDGE ( 'NONE', *, *, #2374, .T. ) ;
#3022=AXIS2_PLACEMENT_3D ( 'NONE', #6723, #856, #3156 ) ;
#3027=DIRECTION ( 'NONE',  ( -5.715354789845005112E-18, -9.999836672264339449E-16, 1.000000000000000000 ) ) ;
#3028=AXIS2_PLACEMENT_3D ( 'NONE', #5238, #6395, #2917 ) ;
#3029=EDGE_LOOP ( 'NONE', ( #1715, #2294, #1630, #2805 ) ) ;
#3030=ORIENTED_EDGE ( 'NONE', *, *, #1540, .T. ) ;
#3031=VECTOR ( 'NONE', #3674, 1000.000000000000000 ) ;
#3037=VECTOR ( 'NONE', #5728, 1000.000000000000000 ) ;
#3040=DIRECTION ( 'NONE',  ( -0.9999836672264333925, 0.005715354789844381486, 0.000000000000000000 ) ) ;
#3042=EDGE_CURVE ( 'NONE', #3635, #3563, #7427, .T. ) ;
#3046=CARTESIAN_POINT ( 'NONE',  ( -7.741417275248890562, 12.33509147838778830, 1.214306433183764966E-14 ) ) ;
#3052=EDGE_CURVE ( 'NONE', #6755, #3946, #661, .T. ) ;
#3054=CARTESIAN_POINT ( 'NONE',  ( 14.29543924104632779, -35.83228874779774742, 2.999999999999964473 ) ) ;
#3056=UNCERTAINTY_MEASURE_WITH_UNIT (LENGTH_MEASURE( 1.000000000000000082E-05 ), #2434, 'distance_accuracy_value', 'NONE');
#3065=CARTESIAN_POINT ( 'NONE',  ( 25.15036705625666258, 26.15624279088186910, 3.000000000000026645 ) ) ;
#3067=ORIENTED_EDGE ( 'NONE', *, *, #3686, .T. ) ;
#3071=CARTESIAN_POINT ( 'NONE',  ( 19.86817077757007510, -41.71399671145089627, 2.999999999999958256 ) ) ;
#3074=ORIENTED_EDGE ( 'NONE', *, *, #3142, .F. ) ;
#3077=B_SPLINE_CURVE_WITH_KNOTS ( 'NONE', 3,
 ( #4830, #5893, #7114, #1955 ),
 .UNSPECIFIED., .F., .F.,
 ( 4, 4 ),
 ( 0.000000000000000000, 1.000000000000000000 ),
 .UNSPECIFIED. ) ;
#3089=EDGE_CURVE ( 'NONE', #6662, #5560, #4662, .T. ) ;
#3090=CARTESIAN_POINT ( 'NONE',  ( -16.56077119915742202, 1.636355435069148490, -2.993845543551538313 ) ) ;
#3091=EDGE_CURVE ( 'NONE', #5062, #1506, #4248, .T. ) ;
#3092=ORIENTED_EDGE ( 'NONE', *, *, #3091, .F. ) ;
#3094=CARTESIAN_POINT ( 'NONE',  ( -34.88460058024266175, 16.28046363954879183, -0.7438455435519999437 ) ) ;
#3095=LINE ( 'NONE', #3065, #3633 ) ;
#3098=EDGE_CURVE ( 'NONE', #2020, #2611, #3527, .T. ) ;
#3099=EDGE_LOOP ( 'NONE', ( #3376, #4204, #962, #5870 ) ) ;
#3102=CARTESIAN_POINT ( 'NONE',  ( 9.998427761233271482, -32.39925913208585939, 2.999999999999967581 ) ) ;
#3103=CARTESIAN_POINT ( 'NONE',  ( -32.92087242456759100, 14.53869105662955796, -2.993845543551514776 ) ) ;
#3104=DIRECTION ( 'NONE',  ( 0.4039838799357100552, 0.9147661038495522590, 1.399039571475124858E-16 ) ) ;
#3107=EDGE_CURVE ( 'NONE', #1377, #5715, #7249, .T. ) ;
#3108=VECTOR ( 'NONE', #3461, 1000.000000000000000 ) ;
#3109=ORIENTED_EDGE ( 'NONE', *, *, #3089, .T. ) ;
#3118=EDGE_CURVE ( 'NONE', #321, #3534, #2193, .T. ) ;
#3121=CARTESIAN_POINT ( 'NONE',  ( 20.29543457672885154, -41.45429371584162226, 2.999999999999958700 ) ) ;
#3122=LINE ( 'NONE', #3237, #755 ) ;
#3130=ADVANCED_FACE ( 'NONE', ( #6316 ), #3439, .F. ) ;
#3139=CIRCLE ( 'NONE', #6878, 0.7499999999999872324 ) ;
#3141=SHAPE_DEFINITION_REPRESENTATION ( #5433, #4460 ) ;
#3142=EDGE_CURVE ( 'NONE', #1377, #5998, #1754, .T. ) ;
#3143=DIRECTION ( 'NONE',  ( 0.8039121061460955397, -0.3550279469270867794, 0.4771587602596085165 ) ) ;
#3144=DIRECTION ( 'NONE',  ( -5.715354789845005112E-18, -9.999836672264339449E-16, 1.000000000000000000 ) ) ;
#3147=ORIENTED_EDGE ( 'NONE', *, *, #404, .T. ) ;
#3149=AXIS2_PLACEMENT_3D ( 'NONE', #6663, #5478, #305 ) ;
#3152=AXIS2_PLACEMENT_3D ( 'NONE', #3559, #2581, #4845 ) ;
#3156=DIRECTION ( 'NONE',  ( 5.715354789845005112E-18, 9.999836672264339449E-16, -1.000000000000000000 ) ) ;
#3157=VECTOR ( 'NONE', #3104, 1000.000000000000000 ) ;
#3163=CARTESIAN_POINT ( 'NONE',  ( 27.98760434640042050, 26.43260972569849443, -1.493845543551990174 ) ) ;
#3164=DIRECTION ( 'NONE',  ( -0.9828140593167951078, 0.1845982795403117438, 1.789781334969680744E-16 ) ) ;
#3167=DIRECTION ( 'NONE',  ( 0.6513146796332659472, 0.5900073775824578037, -0.4771587602596093491 ) ) ;
#3174=LINE ( 'NONE', #3210, #6890 ) ;
#3176=DIRECTION ( 'NONE',  ( 0.9999836672264332815, -0.005715354789845002517, 0.000000000000000000 ) ) ;
#3183=LINE ( 'NONE', #6215, #3522 ) ;
#3184=DIRECTION ( 'NONE',  ( -0.9147661038495521479, 0.4039838799357104993, 5.097713713877666172E-16 ) ) ;
#3185=CARTESIAN_POINT ( 'NONE',  ( 15.26844188666829893, -16.88471001685938333, -1.691355389077386917E-14 ) ) ;
#3187=ORIENTED_EDGE ( 'NONE', *, *, #2697, .T. ) ;
#3190=CARTESIAN_POINT ( 'NONE',  ( 27.65533861039811114, -36.12687000486613442, -3.599551212651874721E-14 ) ) ;
#3194=CARTESIAN_POINT ( 'NONE',  ( -105.7473861751082040, -118.0666774205683822, 2.999999999999881428 ) ) ;
#3196=EDGE_CURVE ( 'NONE', #3216, #3712, #826, .T. ) ;
#3197=ORIENTED_EDGE ( 'NONE', *, *, #2894, .T. ) ;
#3199=FACE_OUTER_BOUND ( 'NONE', #735, .T. ) ;
#3201=PRODUCT_DEFINITION_CONTEXT ( 'detailed design', #3691, 'design' ) ;
#3203=CARTESIAN_POINT ( 'NONE',  ( 14.29543924104632779, -35.83228874779774742, 2.999999999999964473 ) ) ;
#3205=DIRECTION ( 'NONE',  ( 0.3536350175650656014, 0.3203478684871221560, 0.8788171126619651607 ) ) ;
#3207=DIRECTION ( 'NONE',  ( 0.9999836672264335036, -0.005715354789845008589, 0.000000000000000000 ) ) ;
#3209=CARTESIAN_POINT ( 'NONE',  ( -14.63584665781298000, 13.71482652663877566, 1.357730697108428863 ) ) ;
#3210=CARTESIAN_POINT ( 'NONE',  ( 24.99346688245966419, 26.01411140189437177, 0.006154456448490951831 ) ) ;
#3212=DIRECTION ( 'NONE',  ( -5.715354789845005112E-18, -9.999836672264339449E-16, 1.000000000000000000 ) ) ;
#3216=VERTEX_POINT ( 'NONE', #689 ) ;
#3218=DIRECTION ( 'NONE',  ( 2.207673464680433438E-16, -2.241093068000311301E-16, 1.000000000000000000 ) ) ;
#3224=VERTEX_POINT ( 'NONE', #1858 ) ;
#3225=ORIENTED_EDGE ( 'NONE', *, *, #3142, .T. ) ;
#3226=CYLINDRICAL_SURFACE ( 'NONE', #1472, 3.299999999999999378 ) ;
#3228=CIRCLE ( 'NONE', #4200, 5.000000000000000000 ) ;
#3230=LINE ( 'NONE', #2062, #5788 ) ;
#3234=EDGE_CURVE ( 'NONE', #6135, #5520, #1820, .T. ) ;
#3237=CARTESIAN_POINT ( 'NONE',  ( 26.82878048574519525, 24.30342645899339615, 3.000000000000024425 ) ) ;
#3238=CYLINDRICAL_SURFACE ( 'NONE', #488, 20.00000000000000000 ) ;
#3239=PLANE ( 'NONE',  #3651 ) ;
#3240=VECTOR ( 'NONE', #4413, 1000.000000000000000 ) ;
#3244=ORIENTED_EDGE ( 'NONE', *, *, #7010, .T. ) ;
#3247=PLANE ( 'NONE',  #148 ) ;
#3255=CARTESIAN_POINT ( 'NONE',  ( 14.29543924104632779, -35.83228874779774742, -3.556183125752454544E-14 ) ) ;
#3256=PLANE ( 'NONE',  #5706 ) ;
#3259=EDGE_LOOP ( 'NONE', ( #1215, #624 ) ) ;
#3260=AXIS2_PLACEMENT_3D ( 'NONE', #7207, #2117, #998 ) ;
#3261=PLANE ( 'NONE',  #7236 ) ;
#3262=CARTESIAN_POINT ( 'NONE',  ( 16.88097023408849751, 15.29198909576265919, 0.4060579846640053336 ) ) ;
#3264=AXIS2_PLACEMENT_3D ( 'NONE', #1323, #5969, #2449 ) ;
#3266=DIRECTION ( 'NONE',  ( -0.9999836672264333925, 0.005715354789844381486, 0.000000000000000000 ) ) ;
#3268=VECTOR ( 'NONE', #3027, 1000.000000000000000 ) ;
#3275=CARTESIAN_POINT ( 'NONE',  ( 10.46182022341160867, 4.774967812772741738, 3.000000000000004885 ) ) ;
#3277=DIRECTION ( 'NONE',  ( -5.715354789845005112E-18, -9.999836672264339449E-16, 1.000000000000000000 ) ) ;
#3281=AXIS2_PLACEMENT_3D ( 'NONE', #1454, #2623, #4932 ) ;
#3285=CYLINDRICAL_SURFACE ( 'NONE', #4831, 140.0000000000000000 ) ;
#3286=CARTESIAN_POINT ( 'NONE',  ( -12.68712931281627476, 13.22355527668857356, 1.301042606982605321E-14 ) ) ;
#3287=AXIS2_PLACEMENT_3D ( 'NONE', #2349, #1852, #610 ) ;
#3294=VECTOR ( 'NONE', #2773, 1000.000000000000000 ) ;
#3296=ORIENTED_EDGE ( 'NONE', *, *, #3377, .F. ) ;
#3298=B_SPLINE_CURVE_WITH_KNOTS ( 'NONE', 3,
 ( #285, #3209, #3809, #2613 ),
 .UNSPECIFIED., .F., .F.,
 ( 4, 4 ),
 ( 0.000000000000000000, 1.000000000000000000 ),
 .UNSPECIFIED. ) ;
#3299=FACE_OUTER_BOUND ( 'NONE', #6107, .T. ) ;
#3304=ORIENTED_EDGE ( 'NONE', *, *, #4816, .F. ) ;
#3306=CARTESIAN_POINT ( 'NONE',  ( 7.529070345495034289, 16.11642554373086256, 1.604619215278546562E-14 ) ) ;
#3307=PLANE ( 'NONE',  #2555 ) ;
#3311=ORIENTED_EDGE ( 'NONE', *, *, #2546, .T. ) ;
#3312=APPLICATION_CONTEXT ( 'automotive_design' ) ;
#3316=DIRECTION ( 'NONE',  ( 0.9999836672264333925, -0.005715354789844960016, 0.000000000000000000 ) ) ;
#3318=CARTESIAN_POINT ( 'NONE',  ( 26.67188031194815068, 24.16129507000589527, -2.993845543551515664 ) ) ;
#3320=CARTESIAN_POINT ( 'NONE',  ( 14.29543924104632779, -35.83228874779774742, -3.556183125752454544E-14 ) ) ;
#3322=LINE ( 'NONE', #5066, #512 ) ;
#3324=EDGE_CURVE ( 'NONE', #1468, #3587, #3122, .T. ) ;
#3325=EDGE_CURVE ( 'NONE', #6210, #4023, #6157, .T. ) ;
#3329=ORIENTED_EDGE ( 'NONE', *, *, #3003, .T. ) ;
#3331=VERTEX_POINT ( 'NONE', #2677 ) ;
#3333=VERTEX_POINT ( 'NONE', #2106 ) ;
#3338=FACE_OUTER_BOUND ( 'NONE', #918, .T. ) ;
#3342=ORIENTED_EDGE ( 'NONE', *, *, #5235, .F. ) ;
#3343=CARTESIAN_POINT ( 'NONE',  ( 18.47982041150265431, -39.47532202006953383, -3.946495907847236140E-14 ) ) ;
#3347=LINE ( 'NONE', #5739, #3294 ) ;
#3350=ORIENTED_EDGE ( 'NONE', *, *, #491, .F. ) ;
#3353=DIRECTION ( 'NONE',  ( -5.715354789845005112E-18, -9.999836672264339449E-16, 1.000000000000000000 ) ) ;
#3357=VERTEX_POINT ( 'NONE', #3275 ) ;
#3359=ORIENTED_CLOSED_SHELL ( 'NONE', *, #5200, .F. );
#3361=DIRECTION ( 'NONE',  ( -0.9147661038495522590, 0.4039838799357101107, 0.000000000000000000 ) ) ;
#3362=CARTESIAN_POINT ( 'NONE',  ( -15.00216760413269945, 6.625337177075938833, -3.299999999999993161 ) ) ;
#3364=DIRECTION ( 'NONE',  ( 0.6713653717953950162, -0.7411265327553933080, -3.821372782371131388E-16 ) ) ;
#3366=ORIENTED_EDGE ( 'NONE', *, *, #5917, .F. ) ;
#3367=ORIENTED_EDGE ( 'NONE', *, *, #1780, .F. ) ;
#3368=VERTEX_POINT ( 'NONE', #3877 ) ;
#3370=CARTESIAN_POINT ( 'NONE',  ( 24.99346688245966419, 26.01411140189437532, -2.993845543551503674 ) ) ;
#3372=DIRECTION ( 'NONE',  ( -5.715354789845005112E-18, -9.999836672264339449E-16, 1.000000000000000000 ) ) ;
#3376=ORIENTED_EDGE ( 'NONE', *, *, #1392, .F. ) ;
#3377=EDGE_CURVE ( 'NONE', #7172, #3587, #3837, .T. ) ;
#3382=CARTESIAN_POINT ( 'NONE',  ( 22.42915535073480982, 21.39736943723329432, -1.493845543551513444 ) ) ;
#3384=FILL_AREA_STYLE ('',( #43 ) ) ;
#3385=VERTEX_POINT ( 'NONE', #5555 ) ;
#3387=EDGE_CURVE ( 'NONE', #6745, #3216, #6899, .T. ) ;
#3389=CIRCLE ( 'NONE', #1932, 3.750000000000000000 ) ;
#3394=DIRECTION ( 'NONE',  ( 0.4039838799357109433, 0.9147661038495520369, 9.170600743851225078E-16 ) ) ;
#3396=VECTOR ( 'NONE', #5133, 1000.000000000000114 ) ;
#3402=DIRECTION ( 'NONE',  ( 5.715354789845005112E-18, 9.999836672264339449E-16, -1.000000000000000000 ) ) ;
#3405=VECTOR ( 'NONE', #7143, 1000.000000000000000 ) ;
#3410=ORIENTED_EDGE ( 'NONE', *, *, #609, .T. ) ;
#3412=VECTOR ( 'NONE', #6361, 1000.000000000000000 ) ;
#3414=ORIENTED_EDGE ( 'NONE', *, *, #827, .F. ) ;
#3416=FACE_OUTER_BOUND ( 'NONE', #1398, .T. ) ;
#3419=ADVANCED_FACE ( 'NONE', ( #7267 ), #6593, .T. ) ;
#3423=DIRECTION ( 'NONE',  ( -1.850371707708594129E-14, -4.625929269271485795E-14, 1.000000000000000000 ) ) ;
#3424=DIRECTION ( 'NONE',  ( 0.7411265327553918647, 0.6713653717953965705, 6.883823317368281823E-16 ) ) ;
#3426=EDGE_CURVE ( 'NONE', #1547, #3496, #4946, .T. ) ;
#3427=SURFACE_STYLE_USAGE ( .BOTH. , #5699 ) ;
#3429=ORIENTED_EDGE ( 'NONE', *, *, #5654, .F. ) ;
#3437=DIRECTION ( 'NONE',  ( -5.715354789845005112E-18, -9.999836672264339449E-16, 1.000000000000000000 ) ) ;
#3439=CYLINDRICAL_SURFACE ( 'NONE', #4855, 3.299999999999998934 ) ;
#3446=VERTEX_POINT ( 'NONE', #4340 ) ;
#3450=LINE ( 'NONE', #5762, #1837 ) ;
#3456=EDGE_CURVE ( 'NONE', #5486, #4359, #4254, .T. ) ;
#3457=CARTESIAN_POINT ( 'NONE',  ( -105.7473861751082040, -118.0666774205683822, 2.999999999999881428 ) ) ;
#3461=DIRECTION ( 'NONE',  ( -5.715354789845005112E-18, -9.999836672264339449E-16, 1.000000000000000000 ) ) ;
#3462=LINE ( 'NONE', #6370, #3005 ) ;
#3473=DIRECTION ( 'NONE',  ( -0.9999836672264335036, 0.005715354789845003385, 1.110223024625156047E-16 ) ) ;
#3474=DIRECTION ( 'NONE',  ( 0.9999836672264332815, -0.005715354789845002517, 0.000000000000000000 ) ) ;
#3480=VERTEX_POINT ( 'NONE', #1064 ) ;
#3481=CIRCLE ( 'NONE', #2031, 5.000000000000000000 ) ;
#3487=VECTOR ( 'NONE', #6970, 1000.000000000000227 ) ;
#3496=VERTEX_POINT ( 'NONE', #606 ) ;
#3501=DIRECTION ( 'NONE',  ( -5.715354789845005112E-18, -9.999836672264339449E-16, 1.000000000000000000 ) ) ;
#3506=ORIENTED_EDGE ( 'NONE', *, *, #714, .F. ) ;
#3510=FACE_OUTER_BOUND ( 'NONE', #6696, .T. ) ;
#3517=VERTEX_POINT ( 'NONE', #2782 ) ;
#3518=EDGE_CURVE ( 'NONE', #4029, #2611, #1183, .T. ) ;
#3519=ORIENTED_EDGE ( 'NONE', *, *, #3387, .T. ) ;
#3522=VECTOR ( 'NONE', #3218, 1000.000000000000000 ) ;
#3523=CARTESIAN_POINT ( 'NONE',  ( 26.67188031194815068, 24.16129507000589527, -2.993845543551515664 ) ) ;
#3524=CARTESIAN_POINT ( 'NONE',  ( 14.29543924104632779, -35.83228874779774742, 2.999999999999964473 ) ) ;
#3526=CARTESIAN_POINT ( 'NONE',  ( -13.12771516100364799, 4.746262909141762520, 16.32566479563440609 ) ) ;
#3527=CIRCLE ( 'NONE', #4499, 6.300000000000002487 ) ;
#3530=B_SPLINE_CURVE_WITH_KNOTS ( 'NONE', 1,
 ( #5356, #3644 ),
 .UNSPECIFIED., .F., .F.,
 ( 2, 2 ),
 ( 0.000000000000000000, 1.000000000000000000 ),
 .UNSPECIFIED. ) ;
#3534=VERTEX_POINT ( 'NONE', #2227 ) ;
#3541=DIRECTION ( 'NONE',  ( -0.3536350175650657124, -0.3203478684871222115, -0.8788171126619652718 ) ) ;
#3543=CARTESIAN_POINT ( 'NONE',  ( 12.87643844828394535, 18.94962249585221414, -2.729489053861940739 ) ) ;
#3547=DIRECTION ( 'NONE',  ( 0.9999836672264333925, -0.005715354789844381486, 0.000000000000000000 ) ) ;
#3548=ADVANCED_FACE ( 'NONE', ( #4534 ), #2347, .F. ) ;
#3552=CARTESIAN_POINT ( 'NONE',  ( -17.02208700381124729, 2.051506657828173541, 3.000000000000002220 ) ) ;
#3555=B_SPLINE_SURFACE_WITH_KNOTS ( 'NONE', 1, 3, ( 
 ( #3626, #5948, #775, #5498 ),
 ( #6681, #3732, #3286, #5603 ) ),
 .UNSPECIFIED., .F., .F., .F.,
 ( 2, 2 ),
 ( 4, 4 ),
 ( 0.000000000000000000, 1.000000000000000000 ),
 ( 0.000000000000000000, 1.000000000000000000 ),
 .UNSPECIFIED. ) ;
#3559=CARTESIAN_POINT ( 'NONE',  ( -105.7473861751082040, -118.0666774205683822, -1.188285581044112860E-13 ) ) ;
#3563=VERTEX_POINT ( 'NONE', #1103 ) ;
#3564=ADVANCED_FACE ( 'NONE', ( #573 ), #4569, .F. ) ;
#3574=CARTESIAN_POINT ( 'NONE',  ( -19.65288587824389310, 14.48569475295020226, -2.993845543551517441 ) ) ;
#3587=VERTEX_POINT ( 'NONE', #4498 ) ;
#3588=ORIENTED_CLOSED_SHELL ( 'NONE', *, #4472, .F. );
#3589=VERTEX_POINT ( 'NONE', #2893 ) ;
#3591=DIRECTION ( 'NONE',  ( -0.9999836672264335036, 0.005715354789845008589, 0.000000000000000000 ) ) ;
#3597=DIRECTION ( 'NONE',  ( 0.000000000000000000, 0.000000000000000000, 1.000000000000000000 ) ) ;
#3598=DIRECTION ( 'NONE',  ( 0.4039838799357199361, 0.9147661038495479291, 4.432239818696054780E-17 ) ) ;
#3599=CARTESIAN_POINT ( 'NONE',  ( 10.07902270299396008, 17.77910117033601978, 2.236547809770398132 ) ) ;
#3603=FACE_OUTER_BOUND ( 'NONE', #6712, .T. ) ;
#3608=CARTESIAN_POINT ( 'NONE',  ( 13.14859132361182148, 19.41219719266456423, 0.4060579846639996715 ) ) ;
#3609=CARTESIAN_POINT ( 'NONE',  ( -32.92087242456759100, 14.53869105662955619, 0.006154456448484012937 ) ) ;
#3614=FACE_OUTER_BOUND ( 'NONE', #1463, .T. ) ;
#3621=LINE ( 'NONE', #5403, #3985 ) ;
#3624=EDGE_LOOP ( 'NONE', ( #7321, #4860, #259, #2443 ) ) ;
#3625=ORIENTED_EDGE ( 'NONE', *, *, #7316, .F. ) ;
#3626=CARTESIAN_POINT ( 'NONE',  ( -15.07233531785332659, 13.90759097395377886, 2.236547809770393691 ) ) ;
#3631=VECTOR ( 'NONE', #2165, 1000.000000000000000 ) ;
#3632=ORIENTED_EDGE ( 'NONE', *, *, #1951, .T. ) ;
#3633=VECTOR ( 'NONE', #4887, 1000.000000000000114 ) ;
#3634=ORIENTED_EDGE ( 'NONE', *, *, #5545, .T. ) ;
#3635=VERTEX_POINT ( 'NONE', #1948 ) ;
#3639=DIRECTION ( 'NONE',  ( -2.712383034095203713E-15, 1.348591164987489727E-15, -1.000000000000000000 ) ) ;
#3641=AXIS2_PLACEMENT_3D ( 'NONE', #4384, #7303, #1516 ) ;
#3643=AXIS2_PLACEMENT_3D ( 'NONE', #5381, #213, #3591 ) ;
#3644=CARTESIAN_POINT ( 'NONE',  ( 9.018117650298766108, 16.81805756487467107, -0.3999035282154979054 ) ) ;
#3651=AXIS2_PLACEMENT_3D ( 'NONE', #2641, #1550, #4948 ) ;
#3653=EDGE_CURVE ( 'NONE', #3224, #2318, #5538, .T. ) ;
#3656=AXIS2_PLACEMENT_3D ( 'NONE', #5087, #7373, #2851 ) ;
#3657=VERTEX_POINT ( 'NONE', #2486 ) ;
#3658=DIRECTION ( 'NONE',  ( -0.6713653717953944611, 0.7411265327553937521, -9.186864590530470220E-16 ) ) ;
#3659=EDGE_CURVE ( 'NONE', #6227, #2912, #1812, .T. ) ;
#3665=EDGE_LOOP ( 'NONE', ( #3673, #7189, #2890, #1834 ) ) ;
#3666=VERTEX_POINT ( 'NONE', #790 ) ;
#3667=FACE_BOUND ( 'NONE', #2600, .T. ) ;
#3669=DIRECTION ( 'NONE',  ( 0.7411265327553916427, 0.6713653717953966815, 6.883823317368282809E-16 ) ) ;
#3672=ORIENTED_EDGE ( 'NONE', *, *, #5410, .F. ) ;
#3673=ORIENTED_EDGE ( 'NONE', *, *, #2398, .T. ) ;
#3674=DIRECTION ( 'NONE',  ( -0.8748844214391259255, 0.1369338178966306718, -0.4645711771509057897 ) ) ;
#3680=DIRECTION ( 'NONE',  ( 0.9999836672264335036, -0.005715354789845041548, 0.000000000000000000 ) ) ;
#3682=CARTESIAN_POINT ( 'NONE',  ( -31.91091272472834817, 16.82560631625344172, -2.993845543551523214 ) ) ;
#3686=EDGE_CURVE ( 'NONE', #4811, #4478, #4754, .T. ) ;
#3691=APPLICATION_CONTEXT ( 'automotive_design' ) ;
#3694=ORIENTED_EDGE ( 'NONE', *, *, #4570, .F. ) ;
#3695=EDGE_CURVE ( 'NONE', #901, #2204, #5894, .T. ) ;
#3696=EDGE_CURVE ( 'NONE', #216, #909, #2522, .T. ) ;
#3698=EDGE_LOOP ( 'NONE', ( #3798, #5346, #7228, #1724 ) ) ;
#3705=EDGE_CURVE ( 'NONE', #4811, #1688, #7110, .T. ) ;
#3707=ORIENTED_EDGE ( 'NONE', *, *, #4632, .F. ) ;
#3708=DIRECTION ( 'NONE',  ( 0.05111947575938272093, -0.9986925448795970217, -9.983840675197636492E-16 ) ) ;
#3710=CARTESIAN_POINT ( 'NONE',  ( 9.018117650298766108, 16.81805756487467107, -0.3999035282154979054 ) ) ;
#3712=VERTEX_POINT ( 'NONE', #6373 ) ;
#3715=VECTOR ( 'NONE', #7268, 1000.000000000000114 ) ;
#3721=AXIS2_PLACEMENT_3D ( 'NONE', #3090, #1962, #1920 ) ;
#3723=DIRECTION ( 'NONE',  ( 0.7411265327553913096, 0.6713653717953970146, 6.755902076156640294E-16 ) ) ;
#3724=EDGE_CURVE ( 'NONE', #5957, #901, #1324, .T. ) ;
#3726=DIRECTION ( 'NONE',  ( 0.5297244269785086335, 0.8481698128690332572, 8.511835229445635643E-16 ) ) ;
#3731=AXIS2_PLACEMENT_3D ( 'NONE', #3806, #3394, #7306 ) ;
#3732=CARTESIAN_POINT ( 'NONE',  ( -13.25406850835028649, 13.28961593883099468, -0.1384896246987418478 ) ) ;
#3733=CARTESIAN_POINT ( 'NONE',  ( 27.65533861039811114, -36.12687000486602784, -3.001370543551575842 ) ) ;
#3735=EDGE_CURVE ( 'NONE', #6877, #5957, #3228, .T. ) ;
#3737=DIRECTION ( 'NONE',  ( -5.715354789845005112E-18, -9.999836672264339449E-16, 1.000000000000000000 ) ) ;
#3745=FACE_OUTER_BOUND ( 'NONE', #479, .T. ) ;
#3747=PLANE ( 'NONE',  #4873 ) ;
#3752=EDGE_LOOP ( 'NONE', ( #5108, #5628, #5941, #4167 ) ) ;
#3753=CYLINDRICAL_SURFACE ( 'NONE', #4732, 0.7499999999999997780 ) ;
#3762=ORIENTED_EDGE ( 'NONE', *, *, #2215, .F. ) ;
#3763=AXIS2_PLACEMENT_3D ( 'NONE', #3981, #7324, #1050 ) ;
#3765=PLANE ( 'NONE',  #6431 ) ;
#3766=DIRECTION ( 'NONE',  ( -0.9147661038495521479, 0.4039838799357104993, 3.987490689252507167E-16 ) ) ;
#3772=ORIENTED_EDGE ( 'NONE', *, *, #4653, .T. ) ;
#3773=CARTESIAN_POINT ( 'NONE',  ( -95.86211798318534250, -102.0316339954322018, -1.027823659516258203E-13 ) ) ;
#3777=DIRECTION ( 'NONE',  ( -5.715354789845005112E-18, -9.999836672264339449E-16, 1.000000000000000000 ) ) ;
#3779=FACE_OUTER_BOUND ( 'NONE', #2718, .T. ) ;
#3783=ORIENTED_EDGE ( 'NONE', *, *, #2374, .F. ) ;
#3784=EDGE_CURVE ( 'NONE', #553, #5560, #5657, .T. ) ;
#3787=DIRECTION ( 'NONE',  ( -0.9147661038495519259, 0.4039838799357109989, 3.942553354492744024E-16 ) ) ;
#3794=CARTESIAN_POINT ( 'NONE',  ( 41.70778007397900211, -94.98992620957551480, -9.454242944073598665E-14 ) ) ;
#3798=ORIENTED_EDGE ( 'NONE', *, *, #6426, .T. ) ;
#3801=CARTESIAN_POINT ( 'NONE',  ( 3.603225912324908187, 20.45020204625077298, -3.299999999999978950 ) ) ;
#3806=CARTESIAN_POINT ( 'NONE',  ( -17.18648583462957902, 1.679248046991888677, -3.299999999999998046 ) ) ;
#3808=CARTESIAN_POINT ( 'NONE',  ( -19.59526946576633222, 14.55287597139389888, 0.006154456448479242447 ) ) ;
#3809=CARTESIAN_POINT ( 'NONE',  ( -14.19935799777262453, 13.52206207932379023, 0.4789135844464635361 ) ) ;
#3812=CYLINDRICAL_SURFACE ( 'NONE', #7003, 1.100000000000000755 ) ;
#3815=VERTEX_POINT ( 'NONE', #1395 ) ;
#3818=CARTESIAN_POINT ( 'NONE',  ( -19.02833027023232404, 14.48681530925147776, 0.1446440811472397281 ) ) ;
#3819=DIRECTION ( 'NONE',  ( 2.207673464680433438E-16, -2.241093068000311301E-16, 1.000000000000000000 ) ) ;
#3823=ORIENTED_EDGE ( 'NONE', *, *, #4402, .T. ) ;
#3828=CIRCLE ( 'NONE', #595, 2.999999999999999556 ) ;
#3830=ADVANCED_FACE ( 'NONE', ( #5431 ), #266, .T. ) ;
#3836=B_SPLINE_CURVE_WITH_KNOTS ( 'NONE', 3,
 ( #639, #79, #6958, #1653, #1138, #4563 ),
 .UNSPECIFIED., .F., .F.,
 ( 4, 2, 4 ),
 ( 0.000000000000000000, 0.5000000000000000000, 1.000000000000000000 ),
 .UNSPECIFIED. ) ;
#3837=LINE ( 'NONE', #6195, #5347 ) ;
#3846=CARTESIAN_POINT ( 'NONE',  ( 8.411763394295572738, 16.69999280642484507, 3.000000000000017764 ) ) ;
#3847=EDGE_CURVE ( 'NONE', #6538, #418, #3828, .T. ) ;
#3856=DIRECTION ( 'NONE',  ( -5.715354789845005112E-18, -9.999836672264339449E-16, 1.000000000000000000 ) ) ;
#3861=ORIENTED_EDGE ( 'NONE', *, *, #6081, .F. ) ;
#3862=AXIS2_PLACEMENT_3D ( 'NONE', #5862, #6823, #6271 ) ;
#3867=VECTOR ( 'NONE', #3639, 1000.000000000000000 ) ;
#3869=DIRECTION ( 'NONE',  ( 5.715354789845005112E-18, 9.999836672264339449E-16, -1.000000000000000000 ) ) ;
#3872=CIRCLE ( 'NONE', #640, 2.249999999999996891 ) ;
#3877=CARTESIAN_POINT ( 'NONE',  ( -19.52657036150868208, 8.623428025244434636, -2.230393353321900918 ) ) ;
#3881=B_SPLINE_CURVE_WITH_KNOTS ( 'NONE', 3,
 ( #2931, #2479, #4782, #3599 ),
 .UNSPECIFIED., .F., .F.,
 ( 4, 4 ),
 ( 0.000000000000000000, 1.000000000000000000 ),
 .UNSPECIFIED. ) ;
#3885=AXIS2_PLACEMENT_3D ( 'NONE', #6335, #740, #4750 ) ;
#3887=CARTESIAN_POINT ( 'NONE',  ( -12.68640736393857082, 13.22347097710891717, 1.616354215094460922E-14 ) ) ;
#3888=ADVANCED_FACE ( 'NONE', ( #4978 ), #6151, .T. ) ;
#3890=DIRECTION ( 'NONE',  ( 0.4039838799357100552, 0.9147661038495522590, 4.432239818696549050E-17 ) ) ;
#3891=VECTOR ( 'NONE', #5097, 1000.000000000000000 ) ;
#3892=DIRECTION ( 'NONE',  ( -0.9828140593167949968, 0.1845982795403122156, 4.010227384219995304E-16 ) ) ;
#3895=DIRECTION ( 'NONE',  ( -5.715354789845005112E-18, -9.999836672264339449E-16, 1.000000000000000000 ) ) ;
#3896=VECTOR ( 'NONE', #1934, 1000.000000000000000 ) ;
#3898=ORIENTED_EDGE ( 'NONE', *, *, #1540, .F. ) ;
#3900=DIRECTION ( 'NONE',  ( 0.9999836672264332815, -0.005715354789845306094, 0.000000000000000000 ) ) ;
#3906=EDGE_LOOP ( 'NONE', ( #3506, #7400, #4205, #6711 ) ) ;
#3907=ORIENTED_EDGE ( 'NONE', *, *, #4602, .F. ) ;
#3913=CARTESIAN_POINT ( 'NONE',  ( 11.37011796090756555, -1.723489934710175753, -1.734723475976807094E-15 ) ) ;
#3915=EDGE_CURVE ( 'NONE', #3496, #1942, #719, .T. ) ;
#3919=CARTESIAN_POINT ( 'NONE',  ( 31.14423615379030608, -4.720863734206126594, -4.336808689942017736E-15 ) ) ;
#3922=VERTEX_POINT ( 'NONE', #5049 ) ;
#3923=DIRECTION ( 'NONE',  ( 0.9999836672264332815, -0.005715354789847320975, 0.000000000000000000 ) ) ;
#3925=LINE ( 'NONE', #2190, #1610 ) ;
#3929=EDGE_CURVE ( 'NONE', #3331, #1468, #601, .T. ) ;
#3930=CARTESIAN_POINT ( 'NONE',  ( -33.11453295935376673, 14.62421645367269463, 1.431146867680865853E-14 ) ) ;
#3935=ORIENTED_EDGE ( 'NONE', *, *, #7033, .F. ) ;
#3936=ORIENTED_EDGE ( 'NONE', *, *, #3929, .F. ) ;
#3937=CARTESIAN_POINT ( 'NONE',  ( -15.07233531785332659, 13.90759097395377886, 2.236547809770392803 ) ) ;
#3946=VERTEX_POINT ( 'NONE', #6225 ) ;
#3948=DIRECTION ( 'NONE',  ( 0.6513146796332660582, 0.5900073775824583588, -0.4771587602596085165 ) ) ;
#3953=EDGE_LOOP ( 'NONE', ( #5337, #2872, #3311, #208 ) ) ;
#3954=CARTESIAN_POINT ( 'NONE',  ( 1.714606436953501688E-17, 2.999951001679301835E-15, 0.000000000000000000 ) ) ;
#3955=DIRECTION ( 'NONE',  ( -3.426943000455268076E-15, 1.019602848034623186E-15, -1.000000000000000000 ) ) ;
#3956=CARTESIAN_POINT ( 'NONE',  ( -4.418648243523263019, 30.02574454609010601, 2.992397996059992238E-14 ) ) ;
#3958=CARTESIAN_POINT ( 'NONE',  ( 14.63763862841553376, 20.11382921380832656, -1.993845543551509447 ) ) ;
#3960=ORIENTED_EDGE ( 'NONE', *, *, #2769, .F. ) ;
#3961=CARTESIAN_POINT ( 'NONE',  ( -21.54648976118723525, 4.049597505996694657, -2.230393353321905359 ) ) ;
#3963=EDGE_CURVE ( 'NONE', #5506, #320, #2025, .T. ) ;
#3964=DIRECTION ( 'NONE',  ( 0.8856191127862077517, 0.4644123028815776988, 4.694663451788343547E-16 ) ) ;
#3969=DIRECTION ( 'NONE',  ( 0.9999836672264335036, -0.005715354789845041548, 0.000000000000000000 ) ) ;
#3976=CARTESIAN_POINT ( 'NONE',  ( 39.48483786921892857, -95.33781693134928048, -9.497611030973018842E-14 ) ) ;
#3977=ORIENTED_EDGE ( 'NONE', *, *, #971, .T. ) ;
#3978=LINE ( 'NONE', #2361, #4002 ) ;
#3979=DIRECTION ( 'NONE',  ( -0.6713653717953944611, 0.7411265327553937521, 3.821372782371133360E-16 ) ) ;
#3981=CARTESIAN_POINT ( 'NONE',  ( -105.7473861751082040, -118.0666774205683822, -1.188285581044112860E-13 ) ) ;
#3985=VECTOR ( 'NONE', #3205, 1000.000000000000114 ) ;
#3986=CYLINDRICAL_SURFACE ( 'NONE', #4618, 2.249999999999996891 ) ;
#3988=DIRECTION ( 'NONE',  ( 0.6713653717953971256, -0.7411265327553914206, -7.372773368101212272E-16 ) ) ;
#3991=FACE_OUTER_BOUND ( 'NONE', #6497, .T. ) ;
#3992=CIRCLE ( 'NONE', #1582, 0.7500000000000000000 ) ;
#3993=ORIENTED_EDGE ( 'NONE', *, *, #1589, .T. ) ;
#3998=DIRECTION ( 'NONE',  ( 0.4039838799357088894, 0.9147661038495528141, -4.517316048718991978E-16 ) ) ;
#4002=VECTOR ( 'NONE', #5845, 1000.000000000000114 ) ;
#4004=ORIENTED_EDGE ( 'NONE', *, *, #2444, .F. ) ;
#4006=CARTESIAN_POINT ( 'NONE',  ( -24.22739558392570203, 5.420192826457481239, 3.306154456448477497 ) ) ;
#4009=DIRECTION ( 'NONE',  ( -0.9147661038495517039, 0.4039838799357113874, -4.956352788505161098E-15 ) ) ;
#4014=DIRECTION ( 'NONE',  ( -0.4039838799357104993, -0.9147661038495521479, -9.170600743851227050E-16 ) ) ;
#4015=ORIENTED_EDGE ( 'NONE', *, *, #4707, .T. ) ;
#4023=VERTEX_POINT ( 'NONE', #7334 ) ;
#4024=PLANE ( 'NONE',  #3028 ) ;
#4025=FACE_BOUND ( 'NONE', #5561, .T. ) ;
#4029=VERTEX_POINT ( 'NONE', #6894 ) ;
#4034=FACE_OUTER_BOUND ( 'NONE', #490, .T. ) ;
#4036=CARTESIAN_POINT ( 'NONE',  ( -95.86211798318534250, -102.0316339954322018, 2.999999999999897415 ) ) ;
#4037=( LENGTH_UNIT ( ) NAMED_UNIT ( * ) SI_UNIT ( .MILLI., .METRE. ) );
#4045=CARTESIAN_POINT ( 'NONE',  ( 4.492111197601039052, 14.38610368760445546, 1.431146867680865853E-14 ) ) ;
#4046=ORIENTED_EDGE ( 'NONE', *, *, #5966, .F. ) ;
#4047=CYLINDRICAL_SURFACE ( 'NONE', #5436, 147.0000000000000000 ) ;
#4049=DIRECTION ( 'NONE',  ( -0.4039838799357098331, -0.9147661038495523700, -8.673617379884154787E-16 ) ) ;
#4050=CARTESIAN_POINT ( 'NONE',  ( -34.88460058024262622, 16.28046363954885933, -2.243845543551999722 ) ) ;
#4053=DIRECTION ( 'NONE',  ( 0.9147661038495520369, -0.4039838799357104437, -3.987490689252506674E-16 ) ) ;
#4054=ORIENTED_EDGE ( 'NONE', *, *, #4346, .F. ) ;
#4055=ORIENTED_EDGE ( 'NONE', *, *, #5919, .T. ) ;
#4056=VERTEX_POINT ( 'NONE', #1141 ) ;
#4057=LINE ( 'NONE', #3370, #6649 ) ;
#4058=LINE ( 'NONE', #6359, #7365 ) ;
#4060=DIRECTION ( 'NONE',  ( -0.3536350175650657124, -0.3203478684871222115, -0.8788171126619652718 ) ) ;
#4062=ORIENTED_EDGE ( 'NONE', *, *, #3735, .T. ) ;
#4063=DIRECTION ( 'NONE',  ( -5.715354789845005112E-18, -9.999836672264339449E-16, 1.000000000000000000 ) ) ;
#4066=CARTESIAN_POINT ( 'NONE',  ( 26.37580682046979774, 24.48813337504584098, -0.8353469048619511783 ) ) ;
#4067=FACE_OUTER_BOUND ( 'NONE', #4408, .T. ) ;
#4070=ORIENTED_EDGE ( 'NONE', *, *, #1144, .T. ) ;
#4073=EDGE_CURVE ( 'NONE', #1170, #6097, #3481, .T. ) ;
#4076=ORIENTED_EDGE ( 'NONE', *, *, #6582, .F. ) ;
#4079=EDGE_CURVE ( 'NONE', #3333, #6558, #6727, .T. ) ;
#4080=CARTESIAN_POINT ( 'NONE',  ( 28.22862315235815345, 26.16654680453439852, -0.8353469048621777748 ) ) ;
#4084=LINE ( 'NONE', #4164, #7222 ) ;
#4087=ORIENTED_EDGE ( 'NONE', *, *, #381, .T. ) ;
#4089=CARTESIAN_POINT ( 'NONE',  ( -16.40387102536037744, 1.778486824056636939, 3.000000000000001776 ) ) ;
#4093=EDGE_LOOP ( 'NONE', ( #3772, #2119, #5570, #2158 ) ) ;
#4095=ORIENTED_EDGE ( 'NONE', *, *, #198, .T. ) ;
#4096=( NAMED_UNIT ( * ) SI_UNIT ( $, .STERADIAN. ) SOLID_ANGLE_UNIT ( ) );
#4100=DIRECTION ( 'NONE',  ( -0.6713653717954000122, 0.7411265327553888671, 8.673617379884183383E-16 ) ) ;
#4104=AXIS2_PLACEMENT_3D ( 'NONE', #4917, #7198, #6632 ) ;
#4111=ORIENTED_EDGE ( 'NONE', *, *, #2636, .T. ) ;
#4115=CARTESIAN_POINT ( 'NONE',  ( 9.998427761233271482, -32.39925913208585939, 2.999999999999967581 ) ) ;
#4126=ORIENTED_EDGE ( 'NONE', *, *, #1053, .F. ) ;
#4130=DIRECTION ( 'NONE',  ( 5.715354789845005112E-18, 9.999836672264339449E-16, -1.000000000000000000 ) ) ;
#4132=DIRECTION ( 'NONE',  ( -0.9147661038495520369, 0.4039838799357109433, 3.987490689252511604E-16 ) ) ;
#4136=B_SPLINE_CURVE_WITH_KNOTS ( 'NONE', 3,
 ( #117, #3574, #710, #3000, #2704, #6216 ),
 .UNSPECIFIED., .F., .F.,
 ( 4, 2, 4 ),
 ( 0.000000000000000000, 0.5000000000000000000, 1.000000000000000000 ),
 .UNSPECIFIED. ) ;
#4138=AXIS2_PLACEMENT_3D ( 'NONE', #576, #5891, #6907 ) ;
#4140=AXIS2_PLACEMENT_3D ( 'NONE', #3526, #4060, #5196 ) ;
#4142=FACE_OUTER_BOUND ( 'NONE', #6541, .T. ) ;
#4156=ORIENTED_EDGE ( 'NONE', *, *, #252, .T. ) ;
#4164=CARTESIAN_POINT ( 'NONE',  ( -33.11453295935376673, 14.62421645367269107, 3.000000000000014211 ) ) ;
#4167=ORIENTED_EDGE ( 'NONE', *, *, #3196, .F. ) ;
#4169=CARTESIAN_POINT ( 'NONE',  ( -24.29636831944148412, 5.264013524081125439, -2.993845543551514776 ) ) ;
#4173=CARTESIAN_POINT ( 'NONE',  ( 43.95774332523846795, -95.00278575785266355, 2.999999999999905409 ) ) ;
#4175=ORIENTED_EDGE ( 'NONE', *, *, #1718, .T. ) ;
#4179=CARTESIAN_POINT ( 'NONE',  ( 15.04504472124806114, -38.21726078621907874, -3.816391647148975608E-14 ) ) ;
#4186=ORIENTED_EDGE ( 'NONE', *, *, #2776, .F. ) ;
#4187=DIRECTION ( 'NONE',  ( 0.6513146796332690558, 0.5900073775824551392, -0.4771587602596084055 ) ) ;
#4190=CARTESIAN_POINT ( 'NONE',  ( 10.77958151816464216, 24.37277465456891079, 3.306154456448493484 ) ) ;
#4200=AXIS2_PLACEMENT_3D ( 'NONE', #1911, #4220, #6513 ) ;
#4204=ORIENTED_EDGE ( 'NONE', *, *, #2990, .T. ) ;
#4205=ORIENTED_EDGE ( 'NONE', *, *, #935, .T. ) ;
#4206=EDGE_LOOP ( 'NONE', ( #7355, #2837, #1052, #2747 ) ) ;
#4210=LINE ( 'NONE', #5420, #3031 ) ;
#4215=ADVANCED_FACE ( 'NONE', ( #5978 ), #5401, .T. ) ;
#4220=DIRECTION ( 'NONE',  ( 5.715354789845005112E-18, 9.999836672264339449E-16, -1.000000000000000000 ) ) ;
#4222=ORIENTED_EDGE ( 'NONE', *, *, #2636, .F. ) ;
#4228=CARTESIAN_POINT ( 'NONE',  ( -24.29636831944148412, 5.264013524081121886, 0.006154456448480109809 ) ) ;
#4230=CIRCLE ( 'NONE', #980, 0.7499999999999896749 ) ;
#4232=ORIENTED_EDGE ( 'NONE', *, *, #3426, .F. ) ;
#4233=ORIENTED_EDGE ( 'NONE', *, *, #6248, .F. ) ;
#4237=LINE ( 'NONE', #4169, #1719 ) ;
#4239=AXIS2_PLACEMENT_3D ( 'NONE', #3457, #4562, #494 ) ;
#4241=ORIENTED_EDGE ( 'NONE', *, *, #1801, .F. ) ;
#4242=ORIENTED_EDGE ( 'NONE', *, *, #3653, .F. ) ;
#4243=VECTOR ( 'NONE', #288, 1000.000000000000000 ) ;
#4246=VECTOR ( 'NONE', #2761, 1000.000000000000000 ) ;
#4247=DIRECTION ( 'NONE',  ( -0.8174211450113052502, -0.5760405121937228756, -5.807029557109332903E-16 ) ) ;
#4248=CIRCLE ( 'NONE', #5224, 2.249999999999996891 ) ;
#4250=VECTOR ( 'NONE', #7240, 1000.000000000000000 ) ;
#4254=B_SPLINE_CURVE_WITH_KNOTS ( 'NONE', 1,
 ( #2028, #5744 ),
 .UNSPECIFIED., .F., .F.,
 ( 2, 2 ),
 ( 0.000000000000000000, 1.000000000000000000 ),
 .UNSPECIFIED. ) ;
#4255=VECTOR ( 'NONE', #3372, 1000.000000000000000 ) ;
#4266=AXIS2_PLACEMENT_3D ( 'NONE', #3801, #1654, #5169 ) ;
#4277=ORIENTED_EDGE ( 'NONE', *, *, #1928, .F. ) ;
#4279=CARTESIAN_POINT ( 'NONE',  ( -7.741417275248890562, 12.33509147838778475, 3.000000000000011990 ) ) ;
#4280=DIRECTION ( 'NONE',  ( -0.4039838799357114985, -0.9147661038495515928, -8.673617379884191272E-16 ) ) ;
#4287=CARTESIAN_POINT ( 'NONE',  ( 43.95483829995806957, -94.87490738911687060, -3.001370543551634906 ) ) ;
#4295=CARTESIAN_POINT ( 'NONE',  ( 19.86817077757007510, -41.71399671145084653, -4.163336342344337027E-14 ) ) ;
#4302=EDGE_CURVE ( 'NONE', #5560, #3333, #5178, .T. ) ;
#4311=EDGE_LOOP ( 'NONE', ( #6282, #6697, #1676, #3960 ) ) ;
#4312=ADVANCED_FACE ( 'NONE', ( #1627 ), #1065, .F. ) ;
#4313=CARTESIAN_POINT ( 'NONE',  ( 27.65533861039811114, -36.12687000486603495, 2.999999999999964029 ) ) ;
#4314=CARTESIAN_POINT ( 'NONE',  ( 12.40979888490706706, -30.61452125107580713, -3.035766082959412415E-14 ) ) ;
#4321=CARTESIAN_POINT ( 'NONE',  ( -19.59526946576633222, 14.55287597139389888, 0.006154456448479242447 ) ) ;
#4323=CARTESIAN_POINT ( 'NONE',  ( 11.49981217310398485, -0.06572658008321753675, 3.000000000000000000 ) ) ;
#4328=DIRECTION ( 'NONE',  ( 0.9147661038495522590, -0.4039838799357101107, 0.000000000000000000 ) ) ;
#4332=CARTESIAN_POINT ( 'NONE',  ( 15.94457129749017277, -41.07922723232461237, -4.119968255444916849E-14 ) ) ;
#4333=DIRECTION ( 'NONE',  ( -0.8856191127862077517, -0.4644123028815776988, -4.694663451788343547E-16 ) ) ;
#4334=EDGE_CURVE ( 'NONE', #3385, #1522, #464, .T. ) ;
#4339=CARTESIAN_POINT ( 'NONE',  ( 22.09517004029793696, 21.09482167756528526, -1.493845543551514332 ) ) ;
#4340=CARTESIAN_POINT ( 'NONE',  ( 11.49981217310398485, -0.06572658008321453915, 0.000000000000000000 ) ) ;
#4342=DIRECTION ( 'NONE',  ( 0.6713653717953965705, -0.7411265327553918647, -7.095217611944926095E-16 ) ) ;
#4344=ADVANCED_FACE ( 'NONE', ( #947 ), #3238, .F. ) ;
#4346=EDGE_CURVE ( 'NONE', #5242, #3657, #5665, .T. ) ;
#4348=EDGE_LOOP ( 'NONE', ( #3935, #3429 ) ) ;
#4350=CARTESIAN_POINT ( 'NONE',  ( 8.553800617183139110, 16.61347289177635034, -0.1384873327366685780 ) ) ;
#4355=EDGE_CURVE ( 'NONE', #6505, #7060, #2715, .T. ) ;
#4357=EDGE_LOOP ( 'NONE', ( #4769, #268, #667 ) ) ;
#4359=VERTEX_POINT ( 'NONE', #4947 ) ;
#4377=DIRECTION ( 'NONE',  ( -5.715354789845005112E-18, -9.999836672264339449E-16, 1.000000000000000000 ) ) ;
#4380=AXIS2_PLACEMENT_3D ( 'NONE', #3203, #2108, #4915 ) ;
#4384=CARTESIAN_POINT ( 'NONE',  ( 1.714606436953501688E-17, 2.999951001679301835E-15, 0.000000000000000000 ) ) ;
#4386=AXIS2_PLACEMENT_3D ( 'NONE', #1096, #497, #6670 ) ;
#4389=LINE ( 'NONE', #1106, #6042 ) ;
#4391=EDGE_LOOP ( 'NONE', ( #6991, #2199, #2621, #6796 ) ) ;
#4394=PLANE ( 'NONE',  #397 ) ;
#4402=EDGE_CURVE ( 'NONE', #4757, #2710, #5020, .T. ) ;
#4408=EDGE_LOOP ( 'NONE', ( #3762, #4062, #1303, #3898 ) ) ;
#4410=ADVANCED_BREP_SHAPE_REPRESENTATION ( '', ( #4713, #751 ), #2789 ) ;
#4412=DIRECTION ( 'NONE',  ( 5.715354789845005112E-18, 9.999836672264339449E-16, -1.000000000000000000 ) ) ;
#4413=DIRECTION ( 'NONE',  ( -5.715354789845005112E-18, -9.999836672264339449E-16, 1.000000000000000000 ) ) ;
#4419=DIRECTION ( 'NONE',  ( 0.8481698128690331462, -0.5297244269785085224, -5.248681837068071230E-16 ) ) ;
#4422=FACE_OUTER_BOUND ( 'NONE', #1310, .T. ) ;
#4424=CARTESIAN_POINT ( 'NONE',  ( 14.63763862841553376, 20.11382921380833011, -2.993845543551509447 ) ) ;
#4425=CARTESIAN_POINT ( 'NONE',  ( -16.40387102536037744, 1.778486824056639826, 1.734723475976807094E-15 ) ) ;
#4428=CARTESIAN_POINT ( 'NONE',  ( -22.27644891976294161, 9.837844043328900057, 3.306154456448478829 ) ) ;
#4429=DIRECTION ( 'NONE',  ( -0.4950421911735701785, 0.8688689365825380539, 8.521476159766246785E-16 ) ) ;
#4430=ORIENTED_EDGE ( 'NONE', *, *, #15, .F. ) ;
#4433=ORIENTED_EDGE ( 'NONE', *, *, #4653, .F. ) ;
#4439=EDGE_LOOP ( 'NONE', ( #3304, #2525, #4087 ) ) ;
#4440=EDGE_CURVE ( 'NONE', #5957, #5943, #4704, .T. ) ;
#4444=DIRECTION ( 'NONE',  ( -5.715354789845005112E-18, -9.999836672264339449E-16, 1.000000000000000000 ) ) ;
#4446=AXIS2_PLACEMENT_3D ( 'NONE', #2711, #7298, #3424 ) ;
#4450=EDGE_LOOP ( 'NONE', ( #928, #6004 ) ) ;
#4454=DIRECTION ( 'NONE',  ( 0.9999836672264332815, -0.005715354789845002517, 0.000000000000000000 ) ) ;
#4455=VECTOR ( 'NONE', #4333, 1000.000000000000114 ) ;
#4457=CARTESIAN_POINT ( 'NONE',  ( -19.77196556206555655, 3.265922675912619866, 2.236547809770379480 ) ) ;
#4458=ORIENTED_EDGE ( 'NONE', *, *, #3098, .T. ) ;
#4459=DIRECTION ( 'NONE',  ( -5.715354789845005112E-18, -9.999836672264339449E-16, 1.000000000000000000 ) ) ;
#4460=SHAPE_REPRESENTATION ( 'Pliers Right Handle Arm', ( #751 ), #2789 ) ;
#4462=CARTESIAN_POINT ( 'NONE',  ( 10.46182022341160867, 4.774967812772744402, 4.770489558936219510E-15 ) ) ;
#4463=CARTESIAN_POINT ( 'NONE',  ( 12.99837876291259064, -32.41640519645540053, 2.999999999999967581 ) ) ;
#4466=DIRECTION ( 'NONE',  ( -0.9147661038495521479, 0.4039838799357104993, 3.987490689252507167E-16 ) ) ;
#4467=ORIENTED_EDGE ( 'NONE', *, *, #5784, .T. ) ;
#4470=DIRECTION ( 'NONE',  ( 0.9999836672264333925, -0.005715354789844381486, 0.000000000000000000 ) ) ;
#4472=CLOSED_SHELL ( 'NONE', ( #2806, #209, #302 ) ) ;
#4475=PLANE ( 'NONE',  #5462 ) ;
#4476=CARTESIAN_POINT ( 'NONE',  ( 26.13478801451176636, 24.75419629621026019, -1.493845543551509891 ) ) ;
#4478=VERTEX_POINT ( 'NONE', #6414 ) ;
#4486=AXIS2_PLACEMENT_3D ( 'NONE', #3163, #5488, #7192 ) ;
#4489=DIRECTION ( 'NONE',  ( -0.6713653717953972366, 0.7411265327553915316, 8.596159621131687339E-16 ) ) ;
#4495=EDGE_CURVE ( 'NONE', #3331, #4841, #1261, .T. ) ;
#4498=CARTESIAN_POINT ( 'NONE',  ( 12.15447797363371052, 11.01039466689934088, 3.000000000000011546 ) ) ;
#4499=AXIS2_PLACEMENT_3D ( 'NONE', #3362, #1668, #4009 ) ;
#4506=EDGE_LOOP ( 'NONE', ( #1428, #5621, #3067, #6262 ) ) ;
#4513=CARTESIAN_POINT ( 'NONE',  ( 24.99346688245966419, 26.01411140189437532, -2.993845543551503674 ) ) ;
#4516=ORIENTED_EDGE ( 'NONE', *, *, #4570, .T. ) ;
#4528=FACE_OUTER_BOUND ( 'NONE', #4630, .T. ) ;
#4531=ORIENTED_EDGE ( 'NONE', *, *, #3426, .T. ) ;
#4533=DIRECTION ( 'NONE',  ( 5.715354789845005112E-18, 9.999836672264339449E-16, -1.000000000000000000 ) ) ;
#4534=FACE_OUTER_BOUND ( 'NONE', #2159, .T. ) ;
#4535=CARTESIAN_POINT ( 'NONE',  ( 13.19545720709724890, -35.82600185752891520, -3.556183125752454544E-14 ) ) ;
#4541=DIRECTION ( 'NONE',  ( -0.4950421911735701785, 0.8688689365825380539, 8.660254037844390366E-16 ) ) ;
#4544=DIRECTION ( 'NONE',  ( -5.715354789845005112E-18, -9.999836672264339449E-16, 1.000000000000000000 ) ) ;
#4548=VERTEX_POINT ( 'NONE', #6446 ) ;
#4550=VERTEX_POINT ( 'NONE', #2633 ) ;
#4551=ORIENTED_EDGE ( 'NONE', *, *, #6011, .T. ) ;
#4552=DIRECTION ( 'NONE',  ( -0.9999836672264332815, 0.005715354789845002517, 0.000000000000000000 ) ) ;
#4556=CYLINDRICAL_SURFACE ( 'NONE', #6661, 5.000000000000000000 ) ;
#4558=ORIENTED_EDGE ( 'NONE', *, *, #3107, .T. ) ;
#4562=DIRECTION ( 'NONE',  ( 5.715354789845005112E-18, 9.999836672264339449E-16, -1.000000000000000000 ) ) ;
#4563=CARTESIAN_POINT ( 'NONE',  ( 14.63763862841553376, 20.11382921380833011, -2.993845543551509447 ) ) ;
#4564=DIRECTION ( 'NONE',  ( 0.7411265327553895332, 0.6713653717953992350, 6.755902076156661002E-16 ) ) ;
#4566=DIRECTION ( 'NONE',  ( -0.9283625964242117057, 0.005306008274017372239, 0.3716379095795966370 ) ) ;
#4569=PLANE ( 'NONE',  #2688 ) ;
#4570=EDGE_CURVE ( 'NONE', #507, #2611, #7335, .T. ) ;
#4573=CARTESIAN_POINT ( 'NONE',  ( 15.01043771185145381, 6.851040774847841242, 3.000000000000007105 ) ) ;
#4576=DIRECTION ( 'NONE',  ( -0.8688689365825379429, -0.4950421911735701230, -5.000000000000004333E-16 ) ) ;
#4582=LINE ( 'NONE', #2870, #271 ) ;
#4585=VERTEX_POINT ( 'NONE', #1545 ) ;
#4587=AXIS2_PLACEMENT_3D ( 'NONE', #6754, #3895, #3969 ) ;
#4590=ORIENTED_EDGE ( 'NONE', *, *, #1458, .F. ) ;
#4592=EDGE_CURVE ( 'NONE', #3589, #3333, #7299, .T. ) ;
#4593=EDGE_CURVE ( 'NONE', #4811, #7283, #2, .T. ) ;
#4596=CARTESIAN_POINT ( 'NONE',  ( -11.40395268922818062, 1.749910050107414738, 1.734723475976807094E-15 ) ) ;
#4602=EDGE_CURVE ( 'NONE', #3922, #4023, #5015, .T. ) ;
#4605=CARTESIAN_POINT ( 'NONE',  ( -0.2323920193587202254, -101.5535681745463279, -1.014813233446432150E-13 ) ) ;
#4607=ORIENTED_EDGE ( 'NONE', *, *, #3098, .F. ) ;
#4617=ORIENTED_EDGE ( 'NONE', *, *, #5886, .F. ) ;
#4618=AXIS2_PLACEMENT_3D ( 'NONE', #1770, #4063, #6365 ) ;
#4621=CARTESIAN_POINT ( 'NONE',  ( -17.02208700381124729, 2.051506657828176650, 2.168404344971008868E-15 ) ) ;
#4630=EDGE_LOOP ( 'NONE', ( #1302, #687, #938 ) ) ;
#4632=EDGE_CURVE ( 'NONE', #6609, #6505, #5659, .T. ) ;
#4637=DIRECTION ( 'NONE',  ( -0.8688689365825379429, -0.4950421911735701230, -3.889776975374848285E-16 ) ) ;
#4641=AXIS2_PLACEMENT_3D ( 'NONE', #3382, #4564, #598 ) ;
#4648=LINE ( 'NONE', #41, #5836 ) ;
#4650=PRESENTATION_STYLE_ASSIGNMENT (( #3427 ) ) ;
#4652=ORIENTED_EDGE ( 'NONE', *, *, #206, .T. ) ;
#4653=EDGE_CURVE ( 'NONE', #2542, #6227, #1512, .T. ) ;
#4657=CARTESIAN_POINT ( 'NONE',  ( 20.29543457672885154, -41.45429371584162226, 2.999999999999958700 ) ) ;
#4661=DIRECTION ( 'NONE',  ( -0.9147661038495505936, 0.4039838799357137744, 3.987490689252539707E-16 ) ) ;
#4662=LINE ( 'NONE', #6238, #1485 ) ;
#4669=LINE ( 'NONE', #3523, #1603 ) ;
#4670=DIRECTION ( 'NONE',  ( 0.5894575778543340583, -0.6507077505550991070, -0.4786639607048190914 ) ) ;
#4674=ORIENTED_EDGE ( 'NONE', *, *, #1810, .T. ) ;
#4675=CARTESIAN_POINT ( 'NONE',  ( -11.43300101767539623, 1.239551422827351201, 3.000000000000001332 ) ) ;
#4686=EDGE_CURVE ( 'NONE', #2204, #5783, #4940, .T. ) ;
#4688=CARTESIAN_POINT ( 'NONE',  ( 1.714606436953501688E-17, 2.999951001679301835E-15, 0.000000000000000000 ) ) ;
#4690=CARTESIAN_POINT ( 'NONE',  ( 15.04504472124806114, -38.21726078621907874, 2.999999999999961808 ) ) ;
#4704=CIRCLE ( 'NONE', #5303, 11.50000000000000178 ) ;
#4707=EDGE_CURVE ( 'NONE', #418, #7431, #3230, .T. ) ;
#4708=LINE ( 'NONE', #1209, #5697 ) ;
#4709=VECTOR ( 'NONE', #1300, 1000.000000000000227 ) ;
#4713=BREP_WITH_VOIDS ( 'NONE', #1460, ( #3359, #3588 ) );
#4720=ORIENTED_EDGE ( 'NONE', *, *, #2930, .T. ) ;
#4722=CARTESIAN_POINT ( 'NONE',  ( -7.547756740462713054, 12.24956608134464986, 0.006154456448477074043 ) ) ;
#4731=VERTEX_POINT ( 'NONE', #6406 ) ;
#4732=AXIS2_PLACEMENT_3D ( 'NONE', #6037, #4328, #1461 ) ;
#4734=EDGE_LOOP ( 'NONE', ( #1528, #4840, #6720, #1214 ) ) ;
#4737=LINE ( 'NONE', #7027, #5691 ) ;
#4739=VECTOR ( 'NONE', #6547, 1000.000000000000227 ) ;
#4746=VECTOR ( 'NONE', #6218, 1000.000000000000000 ) ;
#4747=CARTESIAN_POINT ( 'NONE',  ( -14.38395162568180652, 6.352317343304402009, 3.000000000000006217 ) ) ;
#4748=DIRECTION ( 'NONE',  ( 0.7411265327553895332, 0.6713653717953992350, 6.755902076156661002E-16 ) ) ;
#4749=VECTOR ( 'NONE', #1175, 1000.000000000000227 ) ;
#4750=DIRECTION ( 'NONE',  ( 0.9999836672264333925, -0.005715354789844381486, 0.000000000000000000 ) ) ;
#4753=CARTESIAN_POINT ( 'NONE',  ( 12.08768627091661330, 18.45115358720316223, -2.230393353321901806 ) ) ;
#4754=LINE ( 'NONE', #118, #4929 ) ;
#4756=ADVANCED_FACE ( 'NONE', ( #3991 ), #1656, .T. ) ;
#4757=VERTEX_POINT ( 'NONE', #1776 ) ;
#4759=DIRECTION ( 'NONE',  ( -5.715354789845005112E-18, -9.999836672264339449E-16, 1.000000000000000000 ) ) ;
#4760=CARTESIAN_POINT ( 'NONE',  ( 19.86817077757007510, -41.71399671145089627, 2.999999999999958256 ) ) ;
#4765=CARTESIAN_POINT ( 'NONE',  ( -27.61161960580294661, 13.06853103689918427, -1.493845543551522104 ) ) ;
#4766=ORIENTED_EDGE ( 'NONE', *, *, #343, .T. ) ;
#4769=ORIENTED_EDGE ( 'NONE', *, *, #1940, .F. ) ;
#4782=CARTESIAN_POINT ( 'NONE',  ( 9.290270525626649345, 17.28063226168697497, 2.735643510310428628 ) ) ;
#4783=LINE ( 'NONE', #4858, #4739 ) ;
#4785=ORIENTED_EDGE ( 'NONE', *, *, #2444, .T. ) ;
#4786=ORIENTED_EDGE ( 'NONE', *, *, #5148, .T. ) ;
#4789=FACE_OUTER_BOUND ( 'NONE', #5504, .T. ) ;
#4793=EDGE_LOOP ( 'NONE', ( #4900, #899, #2366, #2517 ) ) ;
#4803=ORIENTED_EDGE ( 'NONE', *, *, #1546, .F. ) ;
#4804=ORIENTED_EDGE ( 'NONE', *, *, #6257, .F. ) ;
#4806=DIRECTION ( 'NONE',  ( -0.9828140593167951078, 0.1845982795403117438, 1.789781334969680744E-16 ) ) ;
#4811=VERTEX_POINT ( 'NONE', #6301 ) ;
#4815=EDGE_CURVE ( 'NONE', #3922, #212, #2258, .T. ) ;
#4816=EDGE_CURVE ( 'NONE', #5972, #5703, #3462, .T. ) ;
#4823=AXIS2_PLACEMENT_3D ( 'NONE', #6868, #5116, #2726 ) ;
#4827=CARTESIAN_POINT ( 'NONE',  ( -4.418648243523263019, 30.02574454609010601, 2.992397996059992238E-14 ) ) ;
#4830=CARTESIAN_POINT ( 'NONE',  ( 13.14859132361180194, 19.41219719266456423, 0.4060579846640096635 ) ) ;
#4831=AXIS2_PLACEMENT_3D ( 'NONE', #5602, #4459, #3207 ) ;
#4833=LINE ( 'NONE', #5934, #1495 ) ;
#4840=ORIENTED_EDGE ( 'NONE', *, *, #3091, .T. ) ;
#4841=VERTEX_POINT ( 'NONE', #2341 ) ;
#4844=CIRCLE ( 'NONE', #1469, 2.999999999999999556 ) ;
#4845=DIRECTION ( 'NONE',  ( 0.9999836672264335036, -0.005715354789845041548, 0.000000000000000000 ) ) ;
#4848=EDGE_LOOP ( 'NONE', ( #1792, #1494, #373, #832 ) ) ;
#4850=CIRCLE ( 'NONE', #1601, 11.50000000000000178 ) ;
#4851=EDGE_LOOP ( 'NONE', ( #291, #4111, #843, #4095 ) ) ;
#4855=AXIS2_PLACEMENT_3D ( 'NONE', #1157, #6914, #1787 ) ;
#4857=VECTOR ( 'NONE', #3964, 1000.000000000000114 ) ;
#4858=CARTESIAN_POINT ( 'NONE',  ( 8.602313654423408451, 24.43087576540405337, 0.4060579846640144375 ) ) ;
#4860=ORIENTED_EDGE ( 'NONE', *, *, #7284, .T. ) ;
#4865=ORIENTED_EDGE ( 'NONE', *, *, #2646, .T. ) ;
#4868=AXIS2_PLACEMENT_3D ( 'NONE', #1804, #4748, #4100 ) ;
#4873=AXIS2_PLACEMENT_3D ( 'NONE', #1388, #3184, #5509 ) ;
#4878=DIRECTION ( 'NONE',  ( 0.9879743132267128081, 0.1546180985661290141, 1.602621969470799848E-16 ) ) ;
#4887=DIRECTION ( 'NONE',  ( -0.8688689365825379429, -0.4950421911735701230, -5.000000000000004333E-16 ) ) ;
#4892=ORIENTED_EDGE ( 'NONE', *, *, #6192, .F. ) ;
#4900=ORIENTED_EDGE ( 'NONE', *, *, #2556, .F. ) ;
#4903=ORIENTED_EDGE ( 'NONE', *, *, #1939, .F. ) ;
#4906=CARTESIAN_POINT ( 'NONE',  ( -95.86211798318534250, -102.0316339954322018, 2.999999999999897415 ) ) ;
#4910=DIRECTION ( 'NONE',  ( -0.7811859829873639693, -0.4156127062761930113, 0.4658481924037536359 ) ) ;
#4911=ADVANCED_FACE ( 'NONE', ( #1714 ), #2696, .F. ) ;
#4915=DIRECTION ( 'NONE',  ( 0.9999836672264332815, -0.005715354789847320975, 0.000000000000000000 ) ) ;
#4917=CARTESIAN_POINT ( 'NONE',  ( 14.29543924104632779, -35.83228874779774742, -3.556183125752454544E-14 ) ) ;
#4919=ORIENTED_EDGE ( 'NONE', *, *, #5410, .T. ) ;
#4920=EDGE_LOOP ( 'NONE', ( #7248, #7028, #5797 ) ) ;
#4922=ADVANCED_FACE ( 'NONE', ( #6830 ), #5070, .T. ) ;
#4927=ORIENTED_EDGE ( 'NONE', *, *, #1951, .F. ) ;
#4929=VECTOR ( 'NONE', #5393, 1000.000000000000227 ) ;
#4931=CARTESIAN_POINT ( 'NONE',  ( 9.998427761233271482, -32.39925913208585939, -3.252606517456513302E-14 ) ) ;
#4932=DIRECTION ( 'NONE',  ( 0.9999836672264332815, -0.005715354789845002517, 0.000000000000000000 ) ) ;
#4933=LINE ( 'NONE', #6657, #3405 ) ;
#4937=ORIENTED_EDGE ( 'NONE', *, *, #404, .F. ) ;
#4940=CIRCLE ( 'NONE', #6382, 147.0000000000000000 ) ;
#4945=DIRECTION ( 'NONE',  ( -0.9147661038495522590, 0.4039838799357101107, 0.000000000000000000 ) ) ;
#4946=LINE ( 'NONE', #385, #1729 ) ;
#4947=CARTESIAN_POINT ( 'NONE',  ( -12.11759654540111875, 13.15705282150456945, 1.301042606982605321E-14 ) ) ;
#4948=DIRECTION ( 'NONE',  ( -0.005715354789845003385, -0.9999836672264335036, -1.000000000000000472E-15 ) ) ;
#4952=ADVANCED_FACE ( 'NONE', ( #552 ), #6795, .T. ) ;
#4953=ADVANCED_FACE ( 'NONE', ( #4999 ), #516, .F. ) ;
#4956=LINE ( 'NONE', #6131, #2319 ) ;
#4958=CIRCLE ( 'NONE', #1707, 2.999999999999999556 ) ;
#4963=ORIENTED_EDGE ( 'NONE', *, *, #3042, .F. ) ;
#4964=VECTOR ( 'NONE', #6846, 1000.000000000000000 ) ;
#4968=CARTESIAN_POINT ( 'NONE',  ( -16.40387102536037744, 1.778486824056639826, 1.734723475976807094E-15 ) ) ;
#4970=VECTOR ( 'NONE', #399, 1000.000000000000000 ) ;
#4971=AXIS2_PLACEMENT_3D ( 'NONE', #6297, #3988, #1094 ) ;
#4975=DIRECTION ( 'NONE',  ( 0.6713653717953971256, -0.7411265327553914206, -9.593219417351524366E-16 ) ) ;
#4976=AXIS2_PLACEMENT_3D ( 'NONE', #1285, #5306, #3900 ) ;
#4978=FACE_OUTER_BOUND ( 'NONE', #2507, .T. ) ;
#4992=CARTESIAN_POINT ( 'NONE',  ( 25.15036705625666258, 26.15624279088187265, 2.645453300864630819E-14 ) ) ;
#4998=DIRECTION ( 'NONE',  ( -0.9147661038495481511, 0.4039838799357194921, 3.987490689252597393E-16 ) ) ;
#4999=FACE_OUTER_BOUND ( 'NONE', #2821, .T. ) ;
#5001=ORIENTED_EDGE ( 'NONE', *, *, #3963, .F. ) ;
#5002=ORIENTED_EDGE ( 'NONE', *, *, #3325, .T. ) ;
#5006=EDGE_CURVE ( 'NONE', #3368, #4029, #5188, .T. ) ;
#5011=CARTESIAN_POINT ( 'NONE',  ( 21.92563132188826103, 21.95321433679979961, -1.493845543551513444 ) ) ;
#5015=LINE ( 'NONE', #7377, #1809 ) ;
#5018=CARTESIAN_POINT ( 'NONE',  ( -105.7473861751082040, -118.0666774205683822, 2.999999999999881428 ) ) ;
#5020=LINE ( 'NONE', #7304, #604 ) ;
#5023=ORIENTED_EDGE ( 'NONE', *, *, #5235, .T. ) ;
#5028=CARTESIAN_POINT ( 'NONE',  ( 1.714606436953501688E-17, 2.999951001679301835E-15, 0.000000000000000000 ) ) ;
#5032=VERTEX_POINT ( 'NONE', #4765 ) ;
#5036=LINE ( 'NONE', #7320, #3037 ) ;
#5044=CARTESIAN_POINT ( 'NONE',  ( -15.00216760413269945, 6.625337177075936168, 6.505213034913026604E-15 ) ) ;
#5049=CARTESIAN_POINT ( 'NONE',  ( 39.97800414936823188, -95.26063634933134949, -9.497611030973018842E-14 ) ) ;
#5058=CARTESIAN_POINT ( 'NONE',  ( 24.99346688245966419, 26.01411140189437177, 0.006154456448490951831 ) ) ;
#5061=DIRECTION ( 'NONE',  ( 0.6713653717953971256, -0.7411265327553914206, -8.096059920055343791E-16 ) ) ;
#5062=VERTEX_POINT ( 'NONE', #64 ) ;
#5063=CYLINDRICAL_SURFACE ( 'NONE', #6870, 140.0000000000000000 ) ;
#5066=CARTESIAN_POINT ( 'NONE',  ( -27.72086689141953286, 13.93665911791780410, -1.493845543551521216 ) ) ;
#5070=PLANE ( 'NONE',  #840 ) ;
#5077=CARTESIAN_POINT ( 'NONE',  ( -16.40387102536037744, 1.778486824056639826, 1.734723475976807094E-15 ) ) ;
#5087=CARTESIAN_POINT ( 'NONE',  ( 0.000000000000000000, 0.000000000000000000, 3.000000000000000000 ) ) ;
#5095=AXIS2_PLACEMENT_3D ( 'NONE', #1341, #4132, #4280 ) ;
#5097=DIRECTION ( 'NONE',  ( -0.5818022356294096920, 0.8133302887613499399, 8.099917986277619058E-16 ) ) ;
#5101=EDGE_CURVE ( 'NONE', #2020, #1170, #4084, .T. ) ;
#5107=EDGE_LOOP ( 'NONE', ( #6303, #6478, #2127, #920 ) ) ;
#5108=ORIENTED_EDGE ( 'NONE', *, *, #3387, .F. ) ;
#5110=CARTESIAN_POINT ( 'NONE',  ( 25.89376920855426079, 25.02025921737413583, -2.152344182241806347 ) ) ;
#5111=CIRCLE ( 'NONE', #4868, 0.7499999999999872324 ) ;
#5116=DIRECTION ( 'NONE',  ( -0.9180849359830441925, 0.3963837160139272453, 3.911300608320930924E-16 ) ) ;
#5120=ORIENTED_EDGE ( 'NONE', *, *, #2683, .T. ) ;
#5126=CARTESIAN_POINT ( 'NONE',  ( 15.04504472124806114, -38.21726078621907874, -3.816391647148975608E-14 ) ) ;
#5128=VERTEX_POINT ( 'NONE', #6353 ) ;
#5133=DIRECTION ( 'NONE',  ( 0.4364886600403628525, -0.1927644473149890403, -0.8788171126619663820 ) ) ;
#5137=EDGE_LOOP ( 'NONE', ( #4865, #4919, #5869, #10 ) ) ;
#5141=DIRECTION ( 'NONE',  ( -0.4364886600403651840, 0.1927644473149899840, 0.8788171126619650497 ) ) ;
#5146=DIRECTION ( 'NONE',  ( -1.850371707708594129E-14, -4.394632805807911095E-14, 1.000000000000000000 ) ) ;
#5148=EDGE_CURVE ( 'NONE', #5486, #2020, #1272, .T. ) ;
#5150=DIRECTION ( 'NONE',  ( 5.715354789845005112E-18, 9.999836672264339449E-16, -1.000000000000000000 ) ) ;
#5154=ORIENTED_EDGE ( 'NONE', *, *, #3042, .T. ) ;
#5155=ORIENTED_EDGE ( 'NONE', *, *, #1733, .T. ) ;
#5157=ORIENTED_EDGE ( 'NONE', *, *, #5316, .F. ) ;
#5159=CARTESIAN_POINT ( 'NONE',  ( 43.95483829995806957, -94.87490738911687060, -9.454242944073598665E-14 ) ) ;
#5161=CARTESIAN_POINT ( 'NONE',  ( -17.75204616238700339, 7.839753195160374055, 2.236547809770383921 ) ) ;
#5162=CARTESIAN_POINT ( 'NONE',  ( -25.02557223580756585, -4.388903113930568090, -4.336808689942017736E-15 ) ) ;
#5166=ORIENTED_EDGE ( 'NONE', *, *, #1977, .F. ) ;
#5168=PLANE ( 'NONE',  #4971 ) ;
#5169=DIRECTION ( 'NONE',  ( 0.7411265327553913096, 0.6713653717953971256, 6.570922257487902105E-16 ) ) ;
#5173=CARTESIAN_POINT ( 'NONE',  ( -17.48918432324802907, 2.257788664364643871, 3.591483327634216849 ) ) ;
#5177=DIRECTION ( 'NONE',  ( 0.9999836672264332815, -0.005715354789844959149, 0.000000000000000000 ) ) ;
#5178=CIRCLE ( 'NONE', #7083, 20.00000000000000000 ) ;
#5182=DIRECTION ( 'NONE',  ( -0.4039838799357108323, -0.9147661038495518149, -9.170600743851223106E-16 ) ) ;
#5183=VECTOR ( 'NONE', #7265, 1000.000000000000000 ) ;
#5184=CARTESIAN_POINT ( 'NONE',  ( 39.48483786921892857, -95.33781693134928048, -3.001370543551635794 ) ) ;
#5187=ADVANCED_FACE ( 'NONE', ( #2000 ), #5940, .T. ) ;
#5188=LINE ( 'NONE', #6949, #5798 ) ;
#5189=EDGE_CURVE ( 'NONE', #909, #1930, #5374, .T. ) ;
#5191=ORIENTED_EDGE ( 'NONE', *, *, #3324, .T. ) ;
#5194=DIRECTION ( 'NONE',  ( -0.4039838799357112764, -0.9147661038495517039, -1.194615830541411051E-15 ) ) ;
#5196=DIRECTION ( 'NONE',  ( -0.9283625964242117057, 0.005306008274017372239, 0.3716379095795966370 ) ) ;
#5200=CLOSED_SHELL ( 'NONE', ( #5926, #6292, #6416 ) ) ;
#5202=FACE_OUTER_BOUND ( 'NONE', #2001, .T. ) ;
#5204=CARTESIAN_POINT ( 'NONE',  ( 19.34585819626726533, -40.86123582061801329, -4.076600168545496672E-14 ) ) ;
#5205=CARTESIAN_POINT ( 'NONE',  ( 12.08768627091661330, 18.45115358720316223, -2.230393353321891592 ) ) ;
#5207=AXIS2_PLACEMENT_3D ( 'NONE', #4006, #3890, #1156 ) ;
#5208=CIRCLE ( 'NONE', #6407, 2.999999999999999556 ) ;
#5218=CIRCLE ( 'NONE', #3152, 147.0000000000000000 ) ;
#5221=PLANE ( 'NONE',  #2673 ) ;
#5224=AXIS2_PLACEMENT_3D ( 'NONE', #6792, #6865, #6383 ) ;
#5230=DIRECTION ( 'NONE',  ( 0.8039121061460987594, -0.3550279469270790633, 0.4771587602596087385 ) ) ;
#5231=ORIENTED_EDGE ( 'NONE', *, *, #3377, .T. ) ;
#5232=VERTEX_POINT ( 'NONE', #207 ) ;
#5235=EDGE_CURVE ( 'NONE', #3635, #1686, #1692, .T. ) ;
#5238=CARTESIAN_POINT ( 'NONE',  ( -16.21021049057420882, 1.692961427013491615, 0.006154456448471436192 ) ) ;
#5242=VERTEX_POINT ( 'NONE', #1376 ) ;
#5243=AXIS2_PLACEMENT_3D ( 'NONE', #6441, #1874, #2369 ) ;
#5244=ORIENTED_EDGE ( 'NONE', *, *, #5847, .F. ) ;
#5246=EDGE_CURVE ( 'NONE', #6942, #7434, #3621, .T. ) ;
#5250=CARTESIAN_POINT ( 'NONE',  ( 0.000000000000000000, 0.000000000000000000, 3.000000000000000000 ) ) ;
#5254=CARTESIAN_POINT ( 'NONE',  ( 26.73690888918321207, 2.796431673577179922, 3.035766082959412415E-15 ) ) ;
#5271=CYLINDRICAL_SURFACE ( 'NONE', #6646, 5.000000000000000000 ) ;
#5274=ORIENTED_EDGE ( 'NONE', *, *, #2737, .F. ) ;
#5278=CYLINDRICAL_SURFACE ( 'NONE', #5243, 11.50000000000000178 ) ;
#5279=CARTESIAN_POINT ( 'NONE',  ( 41.70778007397900211, -94.98992620957551480, 2.999999999999905409 ) ) ;
#5286=CARTESIAN_POINT ( 'NONE',  ( 14.63763862841555330, 20.11382921380837985, -2.993845543551509447 ) ) ;
#5289=CARTESIAN_POINT ( 'NONE',  ( 15.26844188666829893, -16.88471001685938688, 2.999999999999983125 ) ) ;
#5292=DIRECTION ( 'NONE',  ( -0.4039838799357092780, -0.9147661038495525920, 4.517316048719004797E-16 ) ) ;
#5296=ORIENTED_EDGE ( 'NONE', *, *, #3089, .F. ) ;
#5303=AXIS2_PLACEMENT_3D ( 'NONE', #4688, #7419, #2859 ) ;
#5306=DIRECTION ( 'NONE',  ( -5.715354789845005112E-18, -9.999836672264339449E-16, 1.000000000000000000 ) ) ;
#5308=DIRECTION ( 'NONE',  ( -0.7411265327553895332, -0.6713653717953993461, -1.302304562955136699E-15 ) ) ;
#5314=ADVANCED_FACE ( 'NONE', ( #6596 ), #830, .T. ) ;
#5315=DIRECTION ( 'NONE',  ( 0.7411265327553895332, 0.6713653717953992350, 6.755902076156661002E-16 ) ) ;
#5316=EDGE_CURVE ( 'NONE', #3385, #70, #1577, .T. ) ;
#5322=CIRCLE ( 'NONE', #7113, 147.0000000000000000 ) ;
#5325=CARTESIAN_POINT ( 'NONE',  ( 27.74658554044268399, 26.69867264686258679, -2.152344182241802795 ) ) ;
#5330=CIRCLE ( 'NONE', #6299, 6.300000000000001599 ) ;
#5334=CIRCLE ( 'NONE', #2067, 2.249999999999996891 ) ;
#5335=ORIENTED_EDGE ( 'NONE', *, *, #6919, .F. ) ;
#5337=ORIENTED_EDGE ( 'NONE', *, *, #3705, .F. ) ;
#5338=VECTOR ( 'NONE', #1192, 1000.000000000000000 ) ;
#5339=AXIS2_PLACEMENT_3D ( 'NONE', #6139, #3856, #6072 ) ;
#5345=CARTESIAN_POINT ( 'NONE',  ( 20.29543457672885154, -41.45429371584161515, -3.001370543551582060 ) ) ;
#5346=ORIENTED_EDGE ( 'NONE', *, *, #4602, .T. ) ;
#5347=VECTOR ( 'NONE', #2639, 1000.000000000000227 ) ;
#5350=VERTEX_POINT ( 'NONE', #2643 ) ;
#5351=VECTOR ( 'NONE', #260, 1000.000000000000227 ) ;
#5352=SHAPE_REPRESENTATION_RELATIONSHIP ( 'NONE' , 'NONE' ,  #4460, #4410 ) ;
#5354=DIRECTION ( 'NONE',  ( -0.4039838799357104993, -0.9147661038495521479, -1.912040383129595888E-16 ) ) ;
#5355=AXIS2_PLACEMENT_3D ( 'NONE', #1515, #4945, #3423 ) ;
#5356=CARTESIAN_POINT ( 'NONE',  ( 10.07902270299396008, 17.77910117033601978, 2.236547809770398132 ) ) ;
#5358=CARTESIAN_POINT ( 'NONE',  ( 0.000000000000000000, 0.000000000000000000, 3.000000000000000000 ) ) ;
#5359=EDGE_CURVE ( 'NONE', #7317, #4841, #4389, .T. ) ;
#5361=CARTESIAN_POINT ( 'NONE',  ( 13.75494557961500419, 19.53026195111434404, -2.993845543551520105 ) ) ;
#5366=ADVANCED_FACE ( 'NONE', ( #2183 ), #1520, .T. ) ;
#5367=CARTESIAN_POINT ( 'NONE',  ( 15.01043771185145381, 6.851040774847843906, 6.938893903907228378E-15 ) ) ;
#5374=LINE ( 'NONE', #4228, #1449 ) ;
#5375=EDGE_LOOP ( 'NONE', ( #2506, #1391, #5244, #4467 ) ) ;
#5377=EDGE_CURVE ( 'NONE', #184, #2611, #5711, .T. ) ;
#5380=ORIENTED_EDGE ( 'NONE', *, *, #2398, .F. ) ;
#5381=CARTESIAN_POINT ( 'NONE',  ( -95.86211798318534250, -102.0316339954322018, -1.027823659516258203E-13 ) ) ;
#5382=LINE ( 'NONE', #1968, #6180 ) ;
#5393=DIRECTION ( 'NONE',  ( -0.6713653717953970146, 0.7411265327553913096, 7.633377738797892154E-16 ) ) ;
#5395=ORIENTED_EDGE ( 'NONE', *, *, #4302, .T. ) ;
#5396=DIRECTION ( 'NONE',  ( -0.9147661038495522590, 0.4039838799357101107, 0.000000000000000000 ) ) ;
#5401=CYLINDRICAL_SURFACE ( 'NONE', #122, 6.299999999999997158 ) ;
#5403=CARTESIAN_POINT ( 'NONE',  ( 13.32147353159843028, 12.06754263290683937, -0.3999035282155026794 ) ) ;
#5409=LINE ( 'NONE', #6536, #4243 ) ;
#5410=EDGE_CURVE ( 'NONE', #75, #4478, #1026, .T. ) ;
#5416=ORIENTED_EDGE ( 'NONE', *, *, #3735, .F. ) ;
#5418=VECTOR ( 'NONE', #3277, 1000.000000000000000 ) ;
#5420=CARTESIAN_POINT ( 'NONE',  ( -9.232392015783828398, 12.99354368604250887, 5.337608095967012467 ) ) ;
#5422=FACE_OUTER_BOUND ( 'NONE', #3906, .T. ) ;
#5426=ORIENTED_EDGE ( 'NONE', *, *, #5006, .T. ) ;
#5431=FACE_OUTER_BOUND ( 'NONE', #2003, .T. ) ;
#5433=PRODUCT_DEFINITION_SHAPE ( 'NONE', 'NONE',  #5465 ) ;
#5435=CARTESIAN_POINT ( 'NONE',  ( -28.02385480137100160, 13.25058454003099939, -1.493845543551999944 ) ) ;
#5436=AXIS2_PLACEMENT_3D ( 'NONE', #5716, #3437, #6348 ) ;
#5438=DIRECTION ( 'NONE',  ( -0.7411265327553894222, -0.6713653717953992350, -1.302304562955136501E-15 ) ) ;
#5439=CARTESIAN_POINT ( 'NONE',  ( -30.62055434958606170, 13.52281233407238403, -8.815182418718723767 ) ) ;
#5442=CARTESIAN_POINT ( 'NONE',  ( 18.04796579205319063, 16.34913706177017190, 3.306154456448485490 ) ) ;
#5443=VECTOR ( 'NONE', #6130, 1000.000000000000227 ) ;
#5448=LINE ( 'NONE', #4313, #2301 ) ;
#5449=AXIS2_PLACEMENT_3D ( 'NONE', #3954, #6264, #1102 ) ;
#5450=VECTOR ( 'NONE', #1375, 1000.000000000000000 ) ;
#5454=ORIENTED_EDGE ( 'NONE', *, *, #4495, .T. ) ;
#5458=CIRCLE ( 'NONE', #5339, 3.750000000000000000 ) ;
#5462=AXIS2_PLACEMENT_3D ( 'NONE', #7404, #3979, #5575 ) ;
#5464=DIRECTION ( 'NONE',  ( 0.9999836672264333925, -0.005715354789844381486, 0.000000000000000000 ) ) ;
#5465=PRODUCT_DEFINITION ( 'UNKNOWN', '', #2441, #3201 ) ;
#5473=VECTOR ( 'NONE', #5811, 1000.000000000000000 ) ;
#5476=ADVANCED_FACE ( 'NONE', ( #4422 ), #5668, .T. ) ;
#5478=DIRECTION ( 'NONE',  ( 0.8133302887613500509, 0.5818022356294096920, 5.864412043468331297E-16 ) ) ;
#5480=VECTOR ( 'NONE', #5696, 1000.000000000000000 ) ;
#5486=VERTEX_POINT ( 'NONE', #5600 ) ;
#5488=DIRECTION ( 'NONE',  ( 0.7411265327553895332, 0.6713653717953993461, 1.302304562955136699E-15 ) ) ;
#5495=DIRECTION ( 'NONE',  ( -1.850371707708594129E-14, -4.625929269271485795E-14, 1.000000000000000000 ) ) ;
#5498=CARTESIAN_POINT ( 'NONE',  ( -12.11759654540111875, 13.15705282150456590, 3.000000000000013767 ) ) ;
#5499=DIRECTION ( 'NONE',  ( -5.715354789845005112E-18, -9.999836672264339449E-16, 1.000000000000000000 ) ) ;
#5501=DIRECTION ( 'NONE',  ( -0.4039838799357194921, -0.9147661038495481511, 5.438507216189340937E-17 ) ) ;
#5504=EDGE_LOOP ( 'NONE', ( #4766, #3672, #199, #2055 ) ) ;
#5506=VERTEX_POINT ( 'NONE', #7387 ) ;
#5508=DIRECTION ( 'NONE',  ( 0.4039838799357109433, 0.9147661038495520369, 9.170600743851225078E-16 ) ) ;
#5509=DIRECTION ( 'NONE',  ( 1.153459499832656523E-16, -1.000675586835500184E-15, 1.000000000000000000 ) ) ;
#5517=ADVANCED_FACE ( 'NONE', ( #1663 ), #6269, .T. ) ;
#5518=EDGE_CURVE ( 'NONE', #3357, #1468, #1487, .T. ) ;
#5520=VERTEX_POINT ( 'NONE', #4657 ) ;
#5524=FACE_BOUND ( 'NONE', #4348, .T. ) ;
#5527=ORIENTED_EDGE ( 'NONE', *, *, #5886, .T. ) ;
#5532=DIRECTION ( 'NONE',  ( 0.9999836672264332815, -0.005715354789847320975, 0.000000000000000000 ) ) ;
#5536=ORIENTED_EDGE ( 'NONE', *, *, #1458, .T. ) ;
#5537=ORIENTED_EDGE ( 'NONE', *, *, #5730, .F. ) ;
#5538=CIRCLE ( 'NONE', #2516, 17.99999999999999645 ) ;
#5539=CARTESIAN_POINT ( 'NONE',  ( 15.94457129749017277, -41.07922723232461237, -4.119968255444916849E-14 ) ) ;
#5540=DIRECTION ( 'NONE',  ( 0.9999836672264332815, -0.005715354789845002517, 0.000000000000000000 ) ) ;
#5545=EDGE_CURVE ( 'NONE', #418, #6505, #882, .T. ) ;
#5555=CARTESIAN_POINT ( 'NONE',  ( 13.19545720709724890, -35.82600185752891520, -3.556183125752454544E-14 ) ) ;
#5557=CARTESIAN_POINT ( 'NONE',  ( 20.29543457672885154, -41.45429371584162226, -4.119968255444916849E-14 ) ) ;
#5560=VERTEX_POINT ( 'NONE', #5289 ) ;
#5561=EDGE_LOOP ( 'NONE', ( #1777, #3519 ) ) ;
#5563=LINE ( 'NONE', #4462, #264 ) ;
#5564=CARTESIAN_POINT ( 'NONE',  ( 27.65533861039806496, -36.12687000486608468, -3.599551212651874721E-14 ) ) ;
#5569=ORIENTED_EDGE ( 'NONE', *, *, #827, .T. ) ;
#5570=ORIENTED_EDGE ( 'NONE', *, *, #1939, .T. ) ;
#5571=VECTOR ( 'NONE', #2295, 1000.000000000000000 ) ;
#5574=VECTOR ( 'NONE', #4342, 1000.000000000000114 ) ;
#5575=DIRECTION ( 'NONE',  ( -5.313805496780495629E-16, -9.969792550665913157E-16, 1.000000000000000000 ) ) ;
#5576=CARTESIAN_POINT ( 'NONE',  ( -3.749938752099124972, 0.02143258046192221891, 0.000000000000000000 ) ) ;
#5579=AXIS2_PLACEMENT_3D ( 'NONE', #7133, #1381, #3669 ) ;
#5582=LINE ( 'NONE', #3190, #6061 ) ;
#5583=VECTOR ( 'NONE', #4878, 1000.000000000000114 ) ;
#5600=CARTESIAN_POINT ( 'NONE',  ( -12.11759654540111875, 13.15705282150456590, 3.000000000000012879 ) ) ;
#5601=ORIENTED_EDGE ( 'NONE', *, *, #76, .T. ) ;
#5602=CARTESIAN_POINT ( 'NONE',  ( -95.86211798318534250, -102.0316339954322018, -1.027823659516258203E-13 ) ) ;
#5603=CARTESIAN_POINT ( 'NONE',  ( -12.11759654540111875, 13.15705282150456945, 1.301042606982605321E-14 ) ) ;
#5609=EDGE_CURVE ( 'NONE', #507, #909, #7374, .T. ) ;
#5613=ORIENTED_EDGE ( 'NONE', *, *, #3784, .T. ) ;
#5615=CARTESIAN_POINT ( 'NONE',  ( 28.22862315235815345, 26.16654680453439852, -0.8353469048621777748 ) ) ;
#5617=DIRECTION ( 'NONE',  ( 0.9999836672264333925, -0.005715354789844381486, 0.000000000000000000 ) ) ;
#5619=DIRECTION ( 'NONE',  ( -0.6713653717954000122, 0.7411265327553888671, 8.673617379884183383E-16 ) ) ;
#5621=ORIENTED_EDGE ( 'NONE', *, *, #4593, .F. ) ;
#5624=CARTESIAN_POINT ( 'NONE',  ( -17.64655212076966251, 14.06160472144369500, -1.351576240659936534 ) ) ;
#5628=ORIENTED_EDGE ( 'NONE', *, *, #588, .T. ) ;
#5631=DIRECTION ( 'NONE',  ( 0.6513146796332662802, 0.5900073775824580258, -0.4771587602596085720 ) ) ;
#5637=EDGE_CURVE ( 'NONE', #3224, #1441, #1749, .T. ) ;
#5639=DIRECTION ( 'NONE',  ( -5.715354789845005112E-18, -9.999836672264339449E-16, 1.000000000000000000 ) ) ;
#5645=ORIENTED_EDGE ( 'NONE', *, *, #2071, .F. ) ;
#5652=ORIENTED_EDGE ( 'NONE', *, *, #1669, .T. ) ;
#5654=EDGE_CURVE ( 'NONE', #1522, #4585, #5713, .T. ) ;
#5656=CARTESIAN_POINT ( 'NONE',  ( 19.86817077757007510, -41.71399671145088917, -3.001370543551582060 ) ) ;
#5657=CIRCLE ( 'NONE', #1800, 140.0000000000000000 ) ;
#5659=LINE ( 'NONE', #6775, #5183 ) ;
#5665=LINE ( 'NONE', #5058, #3715 ) ;
#5666=( GEOMETRIC_REPRESENTATION_CONTEXT ( 3 ) GLOBAL_UNCERTAINTY_ASSIGNED_CONTEXT ( ( #722 ) ) GLOBAL_UNIT_ASSIGNED_CONTEXT ( ( #4037, #602, #6338 ) ) REPRESENTATION_CONTEXT ( 'NONE', 'WORKASPACE' ) );
#5668=PLANE ( 'NONE',  #6193 ) ;
#5670=DIRECTION ( 'NONE',  ( -5.715354789845005112E-18, -9.999836672264339449E-16, 1.000000000000000000 ) ) ;
#5674=DIRECTION ( 'NONE',  ( 0.3213584079436493934, -0.3547505615521249767, 0.8779981849197495691 ) ) ;
#5678=ORIENTED_EDGE ( 'NONE', *, *, #2930, .F. ) ;
#5680=VERTEX_POINT ( 'NONE', #6481 ) ;
#5685=CIRCLE ( 'NONE', #622, 3.299999999999999822 ) ;
#5687=LINE ( 'NONE', #5126, #3631 ) ;
#5691=VECTOR ( 'NONE', #2957, 1000.000000000000114 ) ;
#5692=VECTOR ( 'NONE', #1993, 1000.000000000000114 ) ;
#5693=CARTESIAN_POINT ( 'NONE',  ( 8.554393258638587128, 16.61373401801076000, -0.1388209971588536540 ) ) ;
#5694=CARTESIAN_POINT ( 'NONE',  ( -32.59768532061907109, 15.27050393970921327, -1.493845543551520327 ) ) ;
#5696=DIRECTION ( 'NONE',  ( -5.715354789845005112E-18, -9.999836672264339449E-16, 1.000000000000000000 ) ) ;
#5697=VECTOR ( 'NONE', #2289, 1000.000000000000000 ) ;
#5699=SURFACE_SIDE_STYLE ('',( #6963 ) ) ;
#5703=VERTEX_POINT ( 'NONE', #2528 ) ;
#5706=AXIS2_PLACEMENT_3D ( 'NONE', #5077, #6217, #1011 ) ;
#5711=LINE ( 'NONE', #4457, #7226 ) ;
#5712=EDGE_CURVE ( 'NONE', #5715, #1992, #4833, .T. ) ;
#5713=CIRCLE ( 'NONE', #6660, 1.100000000000000755 ) ;
#5715=VERTEX_POINT ( 'NONE', #5325 ) ;
#5716=CARTESIAN_POINT ( 'NONE',  ( -105.7473861751082040, -118.0666774205683822, -1.188285581044112860E-13 ) ) ;
#5718=VECTOR ( 'NONE', #3164, 1000.000000000000227 ) ;
#5721=FACE_OUTER_BOUND ( 'NONE', #929, .T. ) ;
#5728=DIRECTION ( 'NONE',  ( -0.9986925448795970217, -0.05111947575938272093, -5.682652305652042775E-17 ) ) ;
#5730=EDGE_CURVE ( 'NONE', #5520, #6609, #867, .T. ) ;
#5731=DIRECTION ( 'NONE',  ( 0.9999836672264332815, -0.005715354789845306094, 0.000000000000000000 ) ) ;
#5732=DIRECTION ( 'NONE',  ( 0.7411265327553895332, 0.6713653717953992350, 1.304512053934558935E-15 ) ) ;
#5735=DIRECTION ( 'NONE',  ( -0.6713653717954000122, 0.7411265327553888671, 8.673617379884183383E-16 ) ) ;
#5739=CARTESIAN_POINT ( 'NONE',  ( 20.29543457672885154, -41.45429371584161515, -3.001370543551582060 ) ) ;
#5744=CARTESIAN_POINT ( 'NONE',  ( -12.11759654540111875, 13.15705282150456945, 1.301042606982605321E-14 ) ) ;
#5747=DIRECTION ( 'NONE',  ( 5.715354789845005112E-18, 9.999836672264339449E-16, -1.000000000000000000 ) ) ;
#5750=FACE_OUTER_BOUND ( 'NONE', #434, .T. ) ;
#5752=DIRECTION ( 'NONE',  ( 0.7411265327553895332, 0.6713653717953993461, 1.302304562955136699E-15 ) ) ;
#5754=DIRECTION ( 'NONE',  ( 0.9999836672264333925, -0.005715354789844381486, 0.000000000000000000 ) ) ;
#5757=ORIENTED_EDGE ( 'NONE', *, *, #7284, .F. ) ;
#5760=CARTESIAN_POINT ( 'NONE',  ( -34.88460058024266175, 16.28046363954879183, -0.7438455435519999437 ) ) ;
#5762=CARTESIAN_POINT ( 'NONE',  ( -18.46249958194447771, 2.687629333967654244, -0.3999035282155169457 ) ) ;
#5767=EDGE_LOOP ( 'NONE', ( #7165, #1583, #1146, #6429, #4004, #1171, #7356, #2854, #5416, #2566, #4046, #4277, #7388, #4242, #4927, #7402, #7046, #114, #4804, #6955, #2038, #1541, #1048, #4433, #6837, #3367, #1769, #3092, #3625, #2468, #1337, #772, #3414 ) ) ;
#5770=CARTESIAN_POINT ( 'NONE',  ( -31.91091272472834817, 16.82560631625344172, -2.993845543551523214 ) ) ;
#5772=CYLINDRICAL_SURFACE ( 'NONE', #2196, 0.7500000000000003331 ) ;
#5774=DIRECTION ( 'NONE',  ( 0.9571808262218332031, -0.2894907009098718897, -1.790426255900482524E-16 ) ) ;
#5783=VERTEX_POINT ( 'NONE', #165 ) ;
#5784=EDGE_CURVE ( 'NONE', #2318, #4359, #6045, .T. ) ;
#5785=FACE_OUTER_BOUND ( 'NONE', #1196, .T. ) ;
#5786=CYLINDRICAL_SURFACE ( 'NONE', #417, 147.0000000000000000 ) ;
#5787=LINE ( 'NONE', #1072, #4857 ) ;
#5788=VECTOR ( 'NONE', #4377, 1000.000000000000000 ) ;
#5789=DIRECTION ( 'NONE',  ( 0.9147661038495520369, -0.4039838799357104437, -5.652825226190241484E-16 ) ) ;
#5791=LINE ( 'NONE', #17, #5937 ) ;
#5797=ORIENTED_EDGE ( 'NONE', *, *, #1986, .T. ) ;
#5798=VECTOR ( 'NONE', #5230, 1000.000000000000114 ) ;
#5800=ORIENTED_EDGE ( 'NONE', *, *, #175, .T. ) ;
#5801=CARTESIAN_POINT ( 'NONE',  ( 27.98760434640042050, 26.43260972569849443, -1.493845543551990174 ) ) ;
#5809=FACE_OUTER_BOUND ( 'NONE', #219, .T. ) ;
#5810=CYLINDRICAL_SURFACE ( 'NONE', #2344, 0.7500000000000003331 ) ;
#5811=DIRECTION ( 'NONE',  ( -5.715354789845005112E-18, -9.999836672264339449E-16, 1.000000000000000000 ) ) ;
#5812=DIRECTION ( 'NONE',  ( 5.715354789845005112E-18, 9.999836672264339449E-16, -1.000000000000000000 ) ) ;
#5821=DIRECTION ( 'NONE',  ( 3.410558963702386264E-15, 4.255734876089061273E-15, -1.000000000000000000 ) ) ;
#5825=VECTOR ( 'NONE', #3892, 1000.000000000000114 ) ;
#5826=AXIS2_PLACEMENT_3D ( 'NONE', #3255, #7177, #410 ) ;
#5829=DIRECTION ( 'NONE',  ( -5.715354789845005112E-18, -9.999836672264339449E-16, 1.000000000000000000 ) ) ;
#5833=ADVANCED_FACE ( 'NONE', ( #912 ), #346, .F. ) ;
#5836=VECTOR ( 'NONE', #1288, 1000.000000000000000 ) ;
#5840=VERTEX_POINT ( 'NONE', #6811 ) ;
#5845=DIRECTION ( 'NONE',  ( -0.3536350175650626038, -0.3203478684871197690, -0.8788171126619672702 ) ) ;
#5847=EDGE_CURVE ( 'NONE', #2318, #6014, #6258, .T. ) ;
#5853=LINE ( 'NONE', #5770, #150 ) ;
#5854=EDGE_CURVE ( 'NONE', #4023, #321, #7229, .T. ) ;
#5862=CARTESIAN_POINT ( 'NONE',  ( -28.02385480137132845, 13.25058454003066188, -1.493845543551522104 ) ) ;
#5869=ORIENTED_EDGE ( 'NONE', *, *, #2894, .F. ) ;
#5870=ORIENTED_EDGE ( 'NONE', *, *, #310, .F. ) ;
#5873=CARTESIAN_POINT ( 'NONE',  ( 24.99346688245966419, 26.01411140189437532, -2.993845543551503674 ) ) ;
#5874=FACE_OUTER_BOUND ( 'NONE', #3029, .T. ) ;
#5876=LINE ( 'NONE', #2845, #3412 ) ;
#5879=ADVANCED_FACE ( 'NONE', ( #4034 ), #3765, .F. ) ;
#5880=ADVANCED_FACE ( 'NONE', ( #3199 ), #2638, .T. ) ;
#5883=FACE_OUTER_BOUND ( 'NONE', #1564, .T. ) ;
#5886=EDGE_CURVE ( 'NONE', #1686, #3635, #1147, .T. ) ;
#5891=DIRECTION ( 'NONE',  ( 0.4039838799357100552, 0.9147661038495522590, 1.626385516829955012E-16 ) ) ;
#5893=CARTESIAN_POINT ( 'NONE',  ( 13.61290835672744848, 19.61678186576282812, 0.1446417891851695114 ) ) ;
#5894=CIRCLE ( 'NONE', #352, 11.50000000000000178 ) ;
#5901=ORIENTED_EDGE ( 'NONE', *, *, #4707, .F. ) ;
#5911=AXIS2_PLACEMENT_3D ( 'NONE', #917, #800, #5495 ) ;
#5912=ORIENTED_EDGE ( 'NONE', *, *, #77, .T. ) ;
#5917=EDGE_CURVE ( 'NONE', #7060, #5520, #3347, .T. ) ;
#5919=EDGE_CURVE ( 'NONE', #6558, #3357, #2092, .T. ) ;
#5923=FACE_OUTER_BOUND ( 'NONE', #2644, .T. ) ;
#5924=DIRECTION ( 'NONE',  ( 0.9147661038495520369, -0.4039838799357104437, -5.652825226190241484E-16 ) ) ;
#5926=ADVANCED_FACE ( 'NONE', ( #4528 ), #7263, .F. ) ;
#5932=AXIS2_PLACEMENT_3D ( 'NONE', #5367, #2568, #200 ) ;
#5934=CARTESIAN_POINT ( 'NONE',  ( 27.74658554044268399, 26.69867264686258679, -2.152344182241802795 ) ) ;
#5937=VECTOR ( 'NONE', #2909, 1000.000000000000227 ) ;
#5940=PLANE ( 'NONE',  #3721 ) ;
#5941=ORIENTED_EDGE ( 'NONE', *, *, #6240, .T. ) ;
#5943=VERTEX_POINT ( 'NONE', #6849 ) ;
#5945=VERTEX_POINT ( 'NONE', #1694 ) ;
#5946=AXIS2_PLACEMENT_3D ( 'NONE', #2833, #5752, #5674 ) ;
#5947=CIRCLE ( 'NONE', #6068, 5.000000000000000000 ) ;
#5948=CARTESIAN_POINT ( 'NONE',  ( -14.16308857960304302, 13.69107389482846315, 2.735642193797819921 ) ) ;
#5950=AXIS2_PLACEMENT_3D ( 'NONE', #2291, #600, #2888 ) ;
#5955=AXIS2_PLACEMENT_3D ( 'NONE', #9, #5747, #686 ) ;
#5956=ORIENTED_EDGE ( 'NONE', *, *, #1669, .F. ) ;
#5957=VERTEX_POINT ( 'NONE', #567 ) ;
#5959=CARTESIAN_POINT ( 'NONE',  ( 0.000000000000000000, 0.000000000000000000, 0.000000000000000000 ) ) ;
#5961=FACE_OUTER_BOUND ( 'NONE', #1046, .T. ) ;
#5966=EDGE_CURVE ( 'NONE', #427, #5350, #2290, .T. ) ;
#5969=DIRECTION ( 'NONE',  ( -0.9147661038495522590, 0.4039838799357101107, 0.000000000000000000 ) ) ;
#5972=VERTEX_POINT ( 'NONE', #4339 ) ;
#5973=DIRECTION ( 'NONE',  ( 0.4039838799357101107, 0.9147661038495522590, 4.900000000000001209E-14 ) ) ;
#5978=FACE_OUTER_BOUND ( 'NONE', #6766, .T. ) ;
#5981=ORIENTED_EDGE ( 'NONE', *, *, #3696, .F. ) ;
#5982=ORIENTED_EDGE ( 'NONE', *, *, #3705, .T. ) ;
#5983=B_SPLINE_SURFACE_WITH_KNOTS ( 'NONE', 1, 3, ( 
 ( #7287, #2660, #2160, #931 ),
 ( #7214, #4321, #3818, #331 ) ),
 .UNSPECIFIED., .F., .F., .F.,
 ( 2, 2 ),
 ( 4, 4 ),
 ( 0.000000000000000000, 1.000000000000000000 ),
 ( 0.000000000000000000, 1.000000000000000000 ),
 .UNSPECIFIED. ) ;
#5998=VERTEX_POINT ( 'NONE', #4066 ) ;
#6004=ORIENTED_EDGE ( 'NONE', *, *, #6240, .F. ) ;
#6011=EDGE_CURVE ( 'NONE', #7172, #3815, #3881, .T. ) ;
#6013=ADVANCED_FACE ( 'NONE', ( #5961 ), #6960, .T. ) ;
#6014=VERTEX_POINT ( 'NONE', #1210 ) ;
#6016=ORIENTED_EDGE ( 'NONE', *, *, #5377, .T. ) ;
#6017=CARTESIAN_POINT ( 'NONE',  ( 69.23388681508718889, -35.19566595141640875, -3.469446951953614189E-14 ) ) ;
#6024=ORIENTED_EDGE ( 'NONE', *, *, #6641, .T. ) ;
#6030=CARTESIAN_POINT ( 'NONE',  ( -14.38395162568180652, 6.352317343304404673, 6.071532165918824830E-15 ) ) ;
#6034=ORIENTED_EDGE ( 'NONE', *, *, #332, .T. ) ;
#6036=EDGE_LOOP ( 'NONE', ( #7300, #5537, #2801, #280, #2211, #1054, #1554, #174, #4186, #6698, #6281, #4903, #4241, #5613, #5395, #2501, #4055, #6842, #5191, #3296, #2046, #130, #1953, #4786, #778, #467, #3030, #2498, #2790, #328, #4652, #1891, #2373 ) ) ;
#6037=CARTESIAN_POINT ( 'NONE',  ( -34.88460058024264043, 16.28046363954882736, -1.493845543551999944 ) ) ;
#6042=VECTOR ( 'NONE', #7343, 1000.000000000000227 ) ;
#6045=LINE ( 'NONE', #1857, #5718 ) ;
#6046=DIRECTION ( 'NONE',  ( -0.6713653717953970146, 0.7411265327553913096, 7.927884880413787584E-16 ) ) ;
#6053=ORIENTED_EDGE ( 'NONE', *, *, #2071, .T. ) ;
#6056=LINE ( 'NONE', #1442, #5443 ) ;
#6058=AXIS2_PLACEMENT_3D ( 'NONE', #551, #2835, #5754 ) ;
#6059=DIRECTION ( 'NONE',  ( 0.1845982795403122434, 0.9828140593167951078, 2.622080858921231671E-16 ) ) ;
#6061=VECTOR ( 'NONE', #4444, 1000.000000000000000 ) ;
#6065=CONICAL_SURFACE ( 'NONE', #5095, 0.7499999999999865663, 1.029744258676651425 ) ;
#6067=ORIENTED_EDGE ( 'NONE', *, *, #2172, .T. ) ;
#6068=AXIS2_PLACEMENT_3D ( 'NONE', #4089, #6394, #4552 ) ;
#6069=ADVANCED_FACE ( 'NONE', ( #2336 ), #5810, .T. ) ;
#6070=PRODUCT_CONTEXT ( 'NONE', #3312, 'mechanical' ) ;
#6071=ADVANCED_FACE ( 'NONE', ( #2399 ), #5278, .T. ) ;
#6072=DIRECTION ( 'NONE',  ( 0.9999836672264332815, -0.005715354789845002517, 0.000000000000000000 ) ) ;
#6074=DIRECTION ( 'NONE',  ( -5.715354789845005112E-18, -9.999836672264339449E-16, 1.000000000000000000 ) ) ;
#6079=ORIENTED_EDGE ( 'NONE', *, *, #5246, .T. ) ;
#6081=EDGE_CURVE ( 'NONE', #5703, #2927, #5111, .T. ) ;
#6085=DIRECTION ( 'NONE',  ( -0.9999836672264335036, 0.005715354789845008589, 0.000000000000000000 ) ) ;
#6096=LINE ( 'NONE', #7239, #1701 ) ;
#6097=VERTEX_POINT ( 'NONE', #1838 ) ;
#6099=CARTESIAN_POINT ( 'NONE',  ( -7.547756740462723712, 12.24956608134465164, -2.993845543551527655 ) ) ;
#6101=CARTESIAN_POINT ( 'NONE',  ( 14.29543924104632779, -35.83228874779774742, -3.556183125752454544E-14 ) ) ;
#6106=ORIENTED_EDGE ( 'NONE', *, *, #1977, .T. ) ;
#6107=EDGE_LOOP ( 'NONE', ( #1062, #1575, #478, #4015 ) ) ;
#6116=DIRECTION ( 'NONE',  ( -0.9999836672264333925, 0.005715354789844388425, 0.000000000000000000 ) ) ;
#6119=CARTESIAN_POINT ( 'NONE',  ( -31.93002032970718318, 14.10110567601735632, -6.178731080732846159 ) ) ;
#6125=CARTESIAN_POINT ( 'NONE',  ( 5.042816951933372316, 21.20642930254826553, -0.3999035282154982940 ) ) ;
#6129=CARTESIAN_POINT ( 'NONE',  ( 28.12455780688317475, -37.01391159201033076, -3.686287386450715076E-14 ) ) ;
#6130=DIRECTION ( 'NONE',  ( -0.7811859829873639693, -0.4156127062761930113, 0.4658481924037536359 ) ) ;
#6131=CARTESIAN_POINT ( 'NONE',  ( 12.34225220476766438, -34.27182074065601114, -3.426078865054194011E-14 ) ) ;
#6135=VERTEX_POINT ( 'NONE', #3071 ) ;
#6139=CARTESIAN_POINT ( 'NONE',  ( 1.714606436953501688E-17, 2.999951001679301835E-15, 0.000000000000000000 ) ) ;
#6142=LINE ( 'NONE', #7257, #4746 ) ;
#6151=CYLINDRICAL_SURFACE ( 'NONE', #4446, 6.299999999999999822 ) ;
#6152=DIRECTION ( 'NONE',  ( 0.8039121061460987594, -0.3550279469270790633, 0.4771587602596087385 ) ) ;
#6156=EDGE_CURVE ( 'NONE', #6227, #5128, #2098, .T. ) ;
#6157=LINE ( 'NONE', #1997, #5583 ) ;
#6162=AXIS2_PLACEMENT_3D ( 'NONE', #4992, #4541, #7273 ) ;
#6163=DIRECTION ( 'NONE',  ( 5.715354789845005112E-18, 9.999836672264339449E-16, -1.000000000000000000 ) ) ;
#6165=CARTESIAN_POINT ( 'NONE',  ( -7.547756740462723712, 12.24956608134465164, -2.993845543551527655 ) ) ;
#6168=CIRCLE ( 'NONE', #5932, 5.000000000000000000 ) ;
#6169=DIRECTION ( 'NONE',  ( -5.715354789845005112E-18, -9.999836672264339449E-16, 1.000000000000000000 ) ) ;
#6174=CYLINDRICAL_SURFACE ( 'NONE', #528, 3.299999999999999378 ) ;
#6178=CARTESIAN_POINT ( 'NONE',  ( 43.89994888609457035, -93.87291691326068133, -9.367506770274758310E-14 ) ) ;
#6180=VECTOR ( 'NONE', #1307, 1000.000000000000000 ) ;
#6184=CARTESIAN_POINT ( 'NONE',  ( -7.741417275248890562, 12.33509147838778830, 1.214306433183764966E-14 ) ) ;
#6186=AXIS2_PLACEMENT_3D ( 'NONE', #1523, #581, #3474 ) ;
#6187=AXIS2_PLACEMENT_3D ( 'NONE', #5279, #81, #2401 ) ;
#6189=DIRECTION ( 'NONE',  ( 0.9999836672264335036, -0.005715354789845041548, 0.000000000000000000 ) ) ;
#6190=ORIENTED_EDGE ( 'NONE', *, *, #1144, .F. ) ;
#6192=EDGE_CURVE ( 'NONE', #6755, #216, #7141, .T. ) ;
#6193=AXIS2_PLACEMENT_3D ( 'NONE', #3318, #5061, #2829 ) ;
#6195=CARTESIAN_POINT ( 'NONE',  ( 3.875821393968650330, 20.14928133654074927, 3.000000000000020428 ) ) ;
#6200=EDGE_LOOP ( 'NONE', ( #890, #2079, #249, #1133 ) ) ;
#6201=ADVANCED_FACE ( 'NONE', ( #256, #5422 ), #3747, .T. ) ;
#6203=DIRECTION ( 'NONE',  ( 0.9999836672264335036, -0.005715354789845008589, 0.000000000000000000 ) ) ;
#6205=CARTESIAN_POINT ( 'NONE',  ( 13.14859132361180194, 19.41219719266456423, 0.4060579846640096635 ) ) ;
#6210=VERTEX_POINT ( 'NONE', #848 ) ;
#6215=CARTESIAN_POINT ( 'NONE',  ( -31.91091272472834817, 16.82560631625344172, -2.993845543551523214 ) ) ;
#6216=CARTESIAN_POINT ( 'NONE',  ( -17.21006346072928750, 13.86884027412869180, -2.230393353321906247 ) ) ;
#6217=DIRECTION ( 'NONE',  ( 5.715354789845004342E-18, 9.999836672264337477E-16, -1.000000000000000000 ) ) ;
#6218=DIRECTION ( 'NONE',  ( -5.715354789845005112E-18, -9.999836672264339449E-16, 1.000000000000000000 ) ) ;
#6224=CARTESIAN_POINT ( 'NONE',  ( 39.97800414936823188, -95.26063634933134949, 2.999999999999904965 ) ) ;
#6225=CARTESIAN_POINT ( 'NONE',  ( -22.27644891976294161, 9.837844043328894728, -2.993845543551520105 ) ) ;
#6227=VERTEX_POINT ( 'NONE', #222 ) ;
#6228=DIRECTION ( 'NONE',  ( -0.9999836672264335036, 0.005715354789845008589, 0.000000000000000000 ) ) ;
#6235=DIRECTION ( 'NONE',  ( 5.715354789845005112E-18, 9.999836672264339449E-16, -1.000000000000000000 ) ) ;
#6238=CARTESIAN_POINT ( 'NONE',  ( 15.26844188666829893, -16.88471001685938333, -1.691355389077386917E-14 ) ) ;
#6240=EDGE_CURVE ( 'NONE', #5840, #3712, #1267, .T. ) ;
#6244=ORIENTED_EDGE ( 'NONE', *, *, #3052, .T. ) ;
#6248=EDGE_CURVE ( 'NONE', #5350, #1170, #333, .T. ) ;
#6257=EDGE_CURVE ( 'NONE', #3446, #5680, #6783, .T. ) ;
#6258=LINE ( 'NONE', #2027, #5480 ) ;
#6259=AXIS2_PLACEMENT_3D ( 'NONE', #3956, #3353, #3316 ) ;
#6262=ORIENTED_EDGE ( 'NONE', *, *, #343, .F. ) ;
#6264=DIRECTION ( 'NONE',  ( -5.715354789845005112E-18, -9.999836672264339449E-16, 1.000000000000000000 ) ) ;
#6267=MECHANICAL_DESIGN_GEOMETRIC_PRESENTATION_REPRESENTATION('',(#1913),#5666);
#6269=PLANE ( 'NONE',  #3287 ) ;
#6271=DIRECTION ( 'NONE',  ( -0.4039838799357114985, -0.9147661038495515928, -8.673617379884191272E-16 ) ) ;
#6281=ORIENTED_EDGE ( 'NONE', *, *, #3963, .T. ) ;
#6282=ORIENTED_EDGE ( 'NONE', *, *, #1400, .T. ) ;
#6284=CARTESIAN_POINT ( 'NONE',  ( -14.16308857960304302, 13.69107389482846315, 2.735642193797819921 ) ) ;
#6290=EDGE_LOOP ( 'NONE', ( #5757, #139, #3109, #2223 ) ) ;
#6292=ADVANCED_FACE ( 'NONE', ( #2208 ), #1257, .F. ) ;
#6293=LINE ( 'NONE', #5011, #383 ) ;
#6294=EDGE_CURVE ( 'NONE', #4841, #3587, #6880, .T. ) ;
#6296=CARTESIAN_POINT ( 'NONE',  ( 10.77958151816464216, 24.37277465456891079, 3.306154456448493484 ) ) ;
#6297=CARTESIAN_POINT ( 'NONE',  ( 26.82878048574519525, 24.30342645899339971, 2.428612866367529932E-14 ) ) ;
#6299=AXIS2_PLACEMENT_3D ( 'NONE', #2478, #3598, #3143 ) ;
#6301=CARTESIAN_POINT ( 'NONE',  ( 18.04796579205319063, 16.34913706177017545, 0.006154456448481410852 ) ) ;
#6303=ORIENTED_EDGE ( 'NONE', *, *, #3696, .T. ) ;
#6304=VECTOR ( 'NONE', #1112, 1000.000000000000000 ) ;
#6312=ORIENTED_EDGE ( 'NONE', *, *, #7361, .T. ) ;
#6313=DIRECTION ( 'NONE',  ( -0.9147661038495522590, 0.4039838799357101107, 0.000000000000000000 ) ) ;
#6316=FACE_OUTER_BOUND ( 'NONE', #6200, .T. ) ;
#6330=ORIENTED_EDGE ( 'NONE', *, *, #6768, .T. ) ;
#6333=DIRECTION ( 'NONE',  ( 7.436638807346758235E-18, 1.301147106321757529E-15, -1.000000000000000000 ) ) ;
#6334=CARTESIAN_POINT ( 'NONE',  ( -33.11453295935376673, 14.62421645367269463, 1.431146867680865853E-14 ) ) ;
#6335=CARTESIAN_POINT ( 'NONE',  ( 9.998427761233271482, -32.39925913208585939, -3.252606517456513302E-14 ) ) ;
#6338=( NAMED_UNIT ( * ) SI_UNIT ( $, .STERADIAN. ) SOLID_ANGLE_UNIT ( ) );
#6346=DIRECTION ( 'NONE',  ( -5.715354789845005112E-18, -9.999836672264339449E-16, 1.000000000000000000 ) ) ;
#6348=DIRECTION ( 'NONE',  ( 0.9999836672264335036, -0.005715354789845041548, 0.000000000000000000 ) ) ;
#6350=FACE_OUTER_BOUND ( 'NONE', #665, .T. ) ;
#6353=CARTESIAN_POINT ( 'NONE',  ( 27.68174825049008803, -37.24611774345110859, 2.999999999999962697 ) ) ;
#6359=CARTESIAN_POINT ( 'NONE',  ( 26.67188031194815068, 24.16129507000589172, 0.006154456448489217107 ) ) ;
#6361=DIRECTION ( 'NONE',  ( -5.715354789845005112E-18, -9.999836672264339449E-16, 1.000000000000000000 ) ) ;
#6364=ADVANCED_FACE ( 'NONE', ( #484, #4025, #966 ), #3256, .T. ) ;
#6365=DIRECTION ( 'NONE',  ( 0.9999836672264333925, -0.005715354789844388425, 0.000000000000000000 ) ) ;
#6366=CARTESIAN_POINT ( 'NONE',  ( 43.45632180942044442, -94.90042465344848210, 2.999999999999905409 ) ) ;
#6367=CARTESIAN_POINT ( 'NONE',  ( -32.92087242456759100, 14.53869105662955796, -2.993845543551514776 ) ) ;
#6370=CARTESIAN_POINT ( 'NONE',  ( 22.93267937958135860, 20.84152453766674284, -1.493845543551514332 ) ) ;
#6373=CARTESIAN_POINT ( 'NONE',  ( 3.749938752099124972, -0.02143258046191875987, 3.000000000000000000 ) ) ;
#6378=DIRECTION ( 'NONE',  ( -0.9147661038495529251, 0.4039838799357087229, 3.942553354492743531E-16 ) ) ;
#6380=ADVANCED_FACE ( 'NONE', ( #452 ), #4475, .F. ) ;
#6382=AXIS2_PLACEMENT_3D ( 'NONE', #3194, #3869, #6189 ) ;
#6383=DIRECTION ( 'NONE',  ( -0.9999836672264333925, 0.005715354789844388425, 0.000000000000000000 ) ) ;
#6388=ORIENTED_EDGE ( 'NONE', *, *, #2674, .F. ) ;
#6390=ORIENTED_EDGE ( 'NONE', *, *, #1145, .F. ) ;
#6391=VECTOR ( 'NONE', #1740, 1000.000000000000114 ) ;
#6394=DIRECTION ( 'NONE',  ( 5.715354789845005112E-18, 9.999836672264339449E-16, -1.000000000000000000 ) ) ;
#6395=DIRECTION ( 'NONE',  ( -3.872980802086269402E-16, 2.250611045722691657E-16, -1.000000000000000000 ) ) ;
#6397=DIRECTION ( 'NONE',  ( 0.9999836672264332815, -0.005715354789845002517, 0.000000000000000000 ) ) ;
#6399=AXIS2_PLACEMENT_3D ( 'NONE', #1155, #7425, #2381 ) ;
#6404=LINE ( 'NONE', #6442, #5473 ) ;
#6406=CARTESIAN_POINT ( 'NONE',  ( 43.45632180942044442, -94.90042465344848210, -9.454242944073598665E-14 ) ) ;
#6407=AXIS2_PLACEMENT_3D ( 'NONE', #1877, #7170, #3040 ) ;
#6408=AXIS2_PLACEMENT_3D ( 'NONE', #572, #6816, #6228 ) ;
#6414=CARTESIAN_POINT ( 'NONE',  ( 14.63763862841553376, 20.11382921380832656, 0.006154456448485313980 ) ) ;
#6416=ADVANCED_FACE ( 'NONE', ( #3416 ), #1086, .F. ) ;
#6419=CIRCLE ( 'NONE', #5826, 2.500000000000000000 ) ;
#6426=EDGE_CURVE ( 'NONE', #3534, #3922, #2844, .T. ) ;
#6429=ORIENTED_EDGE ( 'NONE', *, *, #1351, .F. ) ;
#6430=ORIENTED_EDGE ( 'NONE', *, *, #6968, .F. ) ;
#6431=AXIS2_PLACEMENT_3D ( 'NONE', #5656, #2819, #6626 ) ;
#6437=EDGE_CURVE ( 'NONE', #5945, #5232, #4648, .T. ) ;
#6440=CYLINDRICAL_SURFACE ( 'NONE', #4976, 2.500000000000000000 ) ;
#6441=CARTESIAN_POINT ( 'NONE',  ( 1.714606436953501688E-17, 2.999951001679301835E-15, 0.000000000000000000 ) ) ;
#6442=CARTESIAN_POINT ( 'NONE',  ( 11.49981217310398485, -0.06572658008321453915, 0.000000000000000000 ) ) ;
#6446=CARTESIAN_POINT ( 'NONE',  ( -27.72086689141922022, 13.93665911791816470, -1.493845543551521216 ) ) ;
#6456=ORIENTED_EDGE ( 'NONE', *, *, #2215, .T. ) ;
#6457=EDGE_LOOP ( 'NONE', ( #7200, #6834, #3329, #2350 ) ) ;
#6459=EDGE_CURVE ( 'NONE', #3446, #6558, #6404, .T. ) ;
#6466=ADVANCED_FACE ( 'NONE', ( #4067 ), #2339, .F. ) ;
#6467=DIRECTION ( 'NONE',  ( 1.000000000000000000, 0.000000000000000000, 0.000000000000000000 ) ) ;
#6473=ADVANCED_FACE ( 'NONE', ( #1738 ), #7038, .F. ) ;
#6475=CARTESIAN_POINT ( 'NONE',  ( 26.13478801451176636, 24.75419629621026019, -1.493845543551509891 ) ) ;
#6478=ORIENTED_EDGE ( 'NONE', *, *, #5189, .T. ) ;
#6481=CARTESIAN_POINT ( 'NONE',  ( 10.46182022341160867, 4.774967812772744402, 4.770489558936219510E-15 ) ) ;
#6486=LINE ( 'NONE', #7054, #5450 ) ;
#6493=FACE_OUTER_BOUND ( 'NONE', #4357, .T. ) ;
#6497=EDGE_LOOP ( 'NONE', ( #6430, #5645, #4232, #5956 ) ) ;
#6498=ADVANCED_FACE ( 'NONE', ( #5883 ), #5772, .T. ) ;
#6501=CARTESIAN_POINT ( 'NONE',  ( -31.91091272472834817, 16.82560631625344172, 0.006154456448481410852 ) ) ;
#6505=VERTEX_POINT ( 'NONE', #5204 ) ;
#6508=VECTOR ( 'NONE', #6235, 1000.000000000000000 ) ;
#6509=DIRECTION ( 'NONE',  ( -1.046706025223848628E-16, 1.111638688234981601E-15, -1.000000000000000000 ) ) ;
#6512=AXIS2_PLACEMENT_3D ( 'NONE', #4425, #6163, #437 ) ;
#6513=DIRECTION ( 'NONE',  ( -0.9999836672264332815, 0.005715354789845002517, 0.000000000000000000 ) ) ;
#6523=AXIS2_PLACEMENT_3D ( 'NONE', #3524, #2281, #5731 ) ;
#6530=ORIENTED_EDGE ( 'NONE', *, *, #3324, .F. ) ;
#6531=EDGE_LOOP ( 'NONE', ( #3350, #4785, #4720, #2161 ) ) ;
#6532=ORIENTED_EDGE ( 'NONE', *, *, #3456, .T. ) ;
#6536=CARTESIAN_POINT ( 'NONE',  ( 43.95483829995806957, -94.87490738911687060, 2.999999999999905409 ) ) ;
#6538=VERTEX_POINT ( 'NONE', #4179 ) ;
#6540=ORIENTED_EDGE ( 'NONE', *, *, #3107, .F. ) ;
#6541=EDGE_LOOP ( 'NONE', ( #1120, #5678, #2657, #1265 ) ) ;
#6543=CARTESIAN_POINT ( 'NONE',  ( -22.27644891976294161, 9.837844043328894728, -2.993845543551559629 ) ) ;
#6544=EDGE_CURVE ( 'NONE', #6210, #6869, #2078, .T. ) ;
#6547=DIRECTION ( 'NONE',  ( -0.6713653717953970146, 0.7411265327553913096, 7.927884880413787584E-16 ) ) ;
#6550=ORIENTED_EDGE ( 'NONE', *, *, #659, .T. ) ;
#6558=VERTEX_POINT ( 'NONE', #4323 ) ;
#6566=ORIENTED_EDGE ( 'NONE', *, *, #4686, .F. ) ;
#6567=ORIENTED_EDGE ( 'NONE', *, *, #2863, .T. ) ;
#6570=ADVANCED_FACE ( 'NONE', ( #2014 ), #299, .T. ) ;
#6577=PLANE ( 'NONE',  #1250 ) ;
#6582=EDGE_CURVE ( 'NONE', #507, #3517, #6614, .T. ) ;
#6583=CARTESIAN_POINT ( 'NONE',  ( -105.7473861751082040, -118.0666774205683822, -1.188285581044112860E-13 ) ) ;
#6589=B_SPLINE_CURVE_WITH_KNOTS ( 'NONE', 3,
 ( #7389, #3808, #2645, #468 ),
 .UNSPECIFIED., .F., .F.,
 ( 4, 4 ),
 ( 0.000000000000000000, 1.000000000000000000 ),
 .UNSPECIFIED. ) ;
#6593=PLANE ( 'NONE',  #1129 ) ;
#6596=FACE_OUTER_BOUND ( 'NONE', #3953, .T. ) ;
#6602=AXIS2_PLACEMENT_3D ( 'NONE', #7187, #6666, #2562 ) ;
#6603=CARTESIAN_POINT ( 'NONE',  ( 7.529070345495034289, 16.11642554373086256, 1.604619215278546562E-14 ) ) ;
#6609=VERTEX_POINT ( 'NONE', #2591 ) ;
#6611=DIRECTION ( 'NONE',  ( -5.715354789845005112E-18, -9.999836672264339449E-16, 1.000000000000000000 ) ) ;
#6612=CARTESIAN_POINT ( 'NONE',  ( 0.000000000000000000, 0.000000000000000000, 3.000000000000000000 ) ) ;
#6614=LINE ( 'NONE', #2624, #3157 ) ;
#6617=ORIENTED_EDGE ( 'NONE', *, *, #1093, .T. ) ;
#6619=FACE_OUTER_BOUND ( 'NONE', #5375, .T. ) ;
#6623=CARTESIAN_POINT ( 'NONE',  ( 9.154985593248634146, -46.96141903535870910, -4.683753385137379155E-14 ) ) ;
#6626=DIRECTION ( 'NONE',  ( 5.715354789845005112E-18, 9.999836672264339449E-16, -1.000000000000000000 ) ) ;
#6632=DIRECTION ( 'NONE',  ( 0.9999836672264332815, -0.005715354789847320975, 0.000000000000000000 ) ) ;
#6633=AXIS2_PLACEMENT_3D ( 'NONE', #6475, #5315, #682 ) ;
#6635=ORIENTED_EDGE ( 'NONE', *, *, #3518, .T. ) ;
#6641=EDGE_CURVE ( 'NONE', #7283, #1942, #4783, .T. ) ;
#6646=AXIS2_PLACEMENT_3D ( 'NONE', #590, #560, #2878 ) ;
#6648=ORIENTED_EDGE ( 'NONE', *, *, #2674, .T. ) ;
#6649=VECTOR ( 'NONE', #1237, 1000.000000000000000 ) ;
#6655=EDGE_CURVE ( 'NONE', #3815, #6686, #3530, .T. ) ;
#6656=CARTESIAN_POINT ( 'NONE',  ( 27.68174825049008803, -37.24611774345110149, -3.001370543551577619 ) ) ;
#6657=CARTESIAN_POINT ( 'NONE',  ( 43.89994888609457035, -93.87291691326068133, -3.001370543551634018 ) ) ;
#6659=ORIENTED_EDGE ( 'NONE', *, *, #1071, .F. ) ;
#6660=AXIS2_PLACEMENT_3D ( 'NONE', #3054, #4759, #1369 ) ;
#6661=AXIS2_PLACEMENT_3D ( 'NONE', #4968, #700, #6397 ) ;
#6662=VERTEX_POINT ( 'NONE', #3185 ) ;
#6663=CARTESIAN_POINT ( 'NONE',  ( 39.97800414936823188, -95.26063634933134949, -3.001370543551635794 ) ) ;
#6666=DIRECTION ( 'NONE',  ( -5.715354789845005112E-18, -9.999836672264339449E-16, 1.000000000000000000 ) ) ;
#6668=ORIENTED_EDGE ( 'NONE', *, *, #749, .T. ) ;
#6670=DIRECTION ( 'NONE',  ( 1.850371707708594760E-14, 4.625929269271487058E-14, -1.000000000000000000 ) ) ;
#6680=EDGE_CURVE ( 'NONE', #6736, #5506, #4933, .T. ) ;
#6681=CARTESIAN_POINT ( 'NONE',  ( -13.76286933773225130, 13.32929763200878881, -0.3999035282155013471 ) ) ;
#6682=DIRECTION ( 'NONE',  ( -0.8688689365825379429, -0.4950421911735701230, -3.889776975374848285E-16 ) ) ;
#6684=DIRECTION ( 'NONE',  ( 0.9999836672264332815, -0.005715354789845002517, 0.000000000000000000 ) ) ;
#6686=VERTEX_POINT ( 'NONE', #3710 ) ;
#6688=ORIENTED_EDGE ( 'NONE', *, *, #1986, .F. ) ;
#6689=VERTEX_POINT ( 'NONE', #257 ) ;
#6696=EDGE_LOOP ( 'NONE', ( #3707, #392, #5901, #3634 ) ) ;
#6697=ORIENTED_EDGE ( 'NONE', *, *, #6966, .T. ) ;
#6698=ORIENTED_EDGE ( 'NONE', *, *, #3003, .F. ) ;
#6704=DIRECTION ( 'NONE',  ( 0.6513146796332652810, 0.5900073775824578037, -0.4771587602596099598 ) ) ;
#6705=ORIENTED_EDGE ( 'NONE', *, *, #4592, .T. ) ;
#6708=FACE_OUTER_BOUND ( 'NONE', #6036, .T. ) ;
#6711=ORIENTED_EDGE ( 'NONE', *, *, #6192, .T. ) ;
#6712=EDGE_LOOP ( 'NONE', ( #4126, #1378, #4070, #6659 ) ) ;
#6713=LINE ( 'NONE', #6017, #4250 ) ;
#6714=FACE_OUTER_BOUND ( 'NONE', #3099, .T. ) ;
#6716=LINE ( 'NONE', #325, #981 ) ;
#6720=ORIENTED_EDGE ( 'NONE', *, *, #2769, .T. ) ;
#6723=CARTESIAN_POINT ( 'NONE',  ( 27.68174825049008803, -37.24611774345110149, -3.001370543551577619 ) ) ;
#6727=CIRCLE ( 'NONE', #599, 11.50000000000000178 ) ;
#6736=VERTEX_POINT ( 'NONE', #6178 ) ;
#6742=DIRECTION ( 'NONE',  ( -0.6713653717953991240, 0.7411265327553895332, 8.112475779533124710E-16 ) ) ;
#6744=CARTESIAN_POINT ( 'NONE',  ( 14.63763862841553376, 20.11382921380833011, -2.993845543551509447 ) ) ;
#6745=VERTEX_POINT ( 'NONE', #5576 ) ;
#6746=CARTESIAN_POINT ( 'NONE',  ( 12.34225220476766438, -34.27182074065601114, -3.426078865054194011E-14 ) ) ;
#6750=AXIS2_PLACEMENT_3D ( 'NONE', #6864, #3361, #2236 ) ;
#6754=CARTESIAN_POINT ( 'NONE',  ( -105.7473861751082040, -118.0666774205683822, -1.188285581044112860E-13 ) ) ;
#6755=VERTEX_POINT ( 'NONE', #2765 ) ;
#6760=ORIENTED_EDGE ( 'NONE', *, *, #3518, .F. ) ;
#6766=EDGE_LOOP ( 'NONE', ( #4531, #770, #2976, #4156 ) ) ;
#6768=EDGE_CURVE ( 'NONE', #5062, #6869, #6142, .T. ) ;
#6774=DIRECTION ( 'NONE',  ( -0.9999836672264335036, 0.005715354789845008589, 0.000000000000000000 ) ) ;
#6775=CARTESIAN_POINT ( 'NONE',  ( 19.34585819626726533, -40.86123582061801329, -4.076600168545496672E-14 ) ) ;
#6778=EDGE_CURVE ( 'NONE', #5943, #89, #1015, .T. ) ;
#6783=CIRCLE ( 'NONE', #3281, 11.50000000000000178 ) ;
#6786=EDGE_LOOP ( 'NONE', ( #1099, #5536, #6532, #1206 ) ) ;
#6787=DIRECTION ( 'NONE',  ( -5.715354789845005112E-18, -9.999836672264339449E-16, 1.000000000000000000 ) ) ;
#6789=EDGE_CURVE ( 'NONE', #1992, #5998, #7260, .T. ) ;
#6792=CARTESIAN_POINT ( 'NONE',  ( 41.70778007397900211, -94.98992620957551480, -9.454242944073598665E-14 ) ) ;
#6794=CYLINDRICAL_SURFACE ( 'NONE', #6058, 2.999999999999999556 ) ;
#6795=PLANE ( 'NONE',  #2764 ) ;
#6796=ORIENTED_EDGE ( 'NONE', *, *, #5101, .F. ) ;
#6801=CARTESIAN_POINT ( 'NONE',  ( 4.492111197601039052, 14.38610368760445191, 3.000000000000014211 ) ) ;
#6811=CARTESIAN_POINT ( 'NONE',  ( -3.749938752099124972, 0.02143258046191922131, 3.000000000000000000 ) ) ;
#6816=DIRECTION ( 'NONE',  ( -5.715354789845005112E-18, -9.999836672264339449E-16, 1.000000000000000000 ) ) ;
#6817=CARTESIAN_POINT ( 'NONE',  ( -15.00216760413269945, 6.625337177075938833, -3.299999999999993161 ) ) ;
#6818=B_SPLINE_CURVE_WITH_KNOTS ( 'NONE', 3,
 ( #1763, #2958, #6952, #1830 ),
 .UNSPECIFIED., .F., .F.,
 ( 4, 4 ),
 ( 0.000000000000000000, 1.000000000000000000 ),
 .UNSPECIFIED. ) ;
#6823=DIRECTION ( 'NONE',  ( -0.9147661038495520369, 0.4039838799357109433, 3.987490689252511604E-16 ) ) ;
#6830=FACE_OUTER_BOUND ( 'NONE', #5137, .T. ) ;
#6834=ORIENTED_EDGE ( 'NONE', *, *, #6680, .T. ) ;
#6837=ORIENTED_EDGE ( 'NONE', *, *, #1589, .F. ) ;
#6842=ORIENTED_EDGE ( 'NONE', *, *, #5518, .T. ) ;
#6845=VECTOR ( 'NONE', #7042, 1000.000000000000114 ) ;
#6846=DIRECTION ( 'NONE',  ( -5.715354789845005112E-18, -9.999836672264339449E-16, 1.000000000000000000 ) ) ;
#6848=DIRECTION ( 'NONE',  ( 0.9999836672264332815, -0.005715354789847320975, 0.000000000000000000 ) ) ;
#6849=CARTESIAN_POINT ( 'NONE',  ( -7.672523287152989369, -8.566351989504937592, -8.673617379884035472E-15 ) ) ;
#6853=EDGE_CURVE ( 'NONE', #6538, #138, #5687, .T. ) ;
#6863=ADVANCED_FACE ( 'NONE', ( #3338 ), #4556, .F. ) ;
#6864=CARTESIAN_POINT ( 'NONE',  ( -28.02385480137100160, 13.25058454003099939, -1.493845543551999944 ) ) ;
#6865=DIRECTION ( 'NONE',  ( -5.715354789845005112E-18, -9.999836672264339449E-16, 1.000000000000000000 ) ) ;
#6868=CARTESIAN_POINT ( 'NONE',  ( 43.45632180942044442, -94.90042465344848210, -3.001370543551634906 ) ) ;
#6869=VERTEX_POINT ( 'NONE', #4173 ) ;
#6870=AXIS2_PLACEMENT_3D ( 'NONE', #3773, #953, #6203 ) ;
#6875=ADVANCED_FACE ( 'NONE', ( #7439 ), #2880, .F. ) ;
#6876=CARTESIAN_POINT ( 'NONE',  ( -13.14279338728291080, 13.42477640308646514, 3.000000000000013323 ) ) ;
#6877=VERTEX_POINT ( 'NONE', #4596 ) ;
#6878=AXIS2_PLACEMENT_3D ( 'NONE', #7155, #7369, #5735 ) ;
#6879=CARTESIAN_POINT ( 'NONE',  ( -4.418648243523263019, 30.02574454609010246, 3.000000000000030198 ) ) ;
#6880=LINE ( 'NONE', #7289, #4255 ) ;
#6885=AXIS2_PLACEMENT_3D ( 'NONE', #7013, #3658, #4187 ) ;
#6889=CARTESIAN_POINT ( 'NONE',  ( -22.27644891976294161, 9.837844043328892951, 0.006154456448479242447 ) ) ;
#6890=VECTOR ( 'NONE', #6682, 1000.000000000000114 ) ;
#6892=AXIS2_PLACEMENT_3D ( 'NONE', #1039, #3364, #1115 ) ;
#6894=CARTESIAN_POINT ( 'NONE',  ( -16.44258018226587836, 7.261459853215404436, -0.3999035282155121718 ) ) ;
#6895=CARTESIAN_POINT ( 'NONE',  ( -14.18862021369882775, 3.785219303680396052, 13.68921345764850450 ) ) ;
#6898=ORIENTED_EDGE ( 'NONE', *, *, #1928, .T. ) ;
#6899=CIRCLE ( 'NONE', #3641, 3.750000000000000000 ) ;
#6900=CIRCLE ( 'NONE', #3643, 140.0000000000000000 ) ;
#6907=DIRECTION ( 'NONE',  ( -0.8039121061460985374, 0.3550279469270785082, -0.4771587602596095712 ) ) ;
#6910=CARTESIAN_POINT ( 'NONE',  ( -32.92087242456759100, 14.53869105662955619, 0.006154456448484012937 ) ) ;
#6914=DIRECTION ( 'NONE',  ( 0.4039838799357096111, 0.9147661038495524810, -1.228182406907795247E-16 ) ) ;
#6918=EDGE_LOOP ( 'NONE', ( #5154, #6106, #842, #3342 ) ) ;
#6919=EDGE_CURVE ( 'NONE', #5943, #2204, #5876, .T. ) ;
#6929=FACE_OUTER_BOUND ( 'NONE', #4734, .T. ) ;
#6933=CARTESIAN_POINT ( 'NONE',  ( -16.40387102536037744, 1.778486824056636939, 3.000000000000001776 ) ) ;
#6942=VERTEX_POINT ( 'NONE', #2430 ) ;
#6944=LINE ( 'NONE', #92, #5351 ) ;
#6949=CARTESIAN_POINT ( 'NONE',  ( -30.62055434958606170, 13.52281233407238403, -8.815182418718723767 ) ) ;
#6951=ORIENTED_EDGE ( 'NONE', *, *, #381, .F. ) ;
#6952=CARTESIAN_POINT ( 'NONE',  ( 7.529070345495034289, 16.11642554373086256, 1.000000000000015987 ) ) ;
#6955=ORIENTED_EDGE ( 'NONE', *, *, #2970, .F. ) ;
#6956=ORIENTED_EDGE ( 'NONE', *, *, #858, .T. ) ;
#6958=CARTESIAN_POINT ( 'NONE',  ( 12.89845119661129758, 18.96985124815245527, -2.671436925771697446 ) ) ;
#6960=PLANE ( 'NONE',  #889 ) ;
#6963=SURFACE_STYLE_FILL_AREA ( #3384 ) ;
#6965=VECTOR ( 'NONE', #5821, 1000.000000000000000 ) ;
#6966=EDGE_CURVE ( 'NONE', #4731, #1000, #316, .T. ) ;
#6968=EDGE_CURVE ( 'NONE', #6686, #6942, #2075, .T. ) ;
#6969=DIRECTION ( 'NONE',  ( 0.9999836672264332815, -0.005715354789845002517, 0.000000000000000000 ) ) ;
#6970=DIRECTION ( 'NONE',  ( 0.7411265327553913096, 0.6713653717953970146, 6.755902076156640294E-16 ) ) ;
#6974=LINE ( 'NONE', #3961, #736 ) ;
#6975=ADVANCED_FACE ( 'NONE', ( #1434 ), #7196, .F. ) ;
#6977=DIRECTION ( 'NONE',  ( -5.715354789845005112E-18, -9.999836672264339449E-16, 1.000000000000000000 ) ) ;
#6983=EDGE_LOOP ( 'NONE', ( #4054, #363, #3823, #2953 ) ) ;
#6991=ORIENTED_EDGE ( 'NONE', *, *, #77, .F. ) ;
#7003=AXIS2_PLACEMENT_3D ( 'NONE', #6101, #3212, #5532 ) ;
#7007=AXIS2_PLACEMENT_3D ( 'NONE', #6879, #1125, #2807 ) ;
#7008=VECTOR ( 'NONE', #4806, 1000.000000000000227 ) ;
#7010=EDGE_CURVE ( 'NONE', #7434, #7283, #2473, .T. ) ;
#7013=CARTESIAN_POINT ( 'NONE',  ( 18.04796579205319063, 16.34913706177017190, 3.306154456448485490 ) ) ;
#7027=CARTESIAN_POINT ( 'NONE',  ( 24.80820526761568345, 22.47304504285837368, -8.815182418718737978 ) ) ;
#7028=ORIENTED_EDGE ( 'NONE', *, *, #1940, .T. ) ;
#7033=EDGE_CURVE ( 'NONE', #4585, #1522, #534, .T. ) ;
#7034=ORIENTED_EDGE ( 'NONE', *, *, #2598, .T. ) ;
#7038=CYLINDRICAL_SURFACE ( 'NONE', #3885, 2.999999999999999556 ) ;
#7042=DIRECTION ( 'NONE',  ( -0.02358931830619094214, 0.9997217333147505602, 9.995705837626804294E-16 ) ) ;
#7046=ORIENTED_EDGE ( 'NONE', *, *, #4495, .F. ) ;
#7048=CARTESIAN_POINT ( 'NONE',  ( 23.12979183812720407, 24.32586137474685017, -8.815182418718713109 ) ) ;
#7051=ADVANCED_FACE ( 'NONE', ( #5524, #2607, #6708 ), #3239, .F. ) ;
#7054=CARTESIAN_POINT ( 'NONE',  ( 26.67188031194815068, 24.16129507000589527, -2.993845543551515664 ) ) ;
#7060=VERTEX_POINT ( 'NONE', #5557 ) ;
#7061=DIRECTION ( 'NONE',  ( -0.005715354789845003385, -0.9999836672264335036, -2.228438827623913869E-16 ) ) ;
#7063=ADVANCED_FACE ( 'NONE', ( #3510 ), #5786, .F. ) ;
#7073=CARTESIAN_POINT ( 'NONE',  ( 14.12411727399747186, 19.86467175049790868, 0.006154456448484880299 ) ) ;
#7077=EDGE_LOOP ( 'NONE', ( #625, #1760, #242, #6550 ) ) ;
#7083=AXIS2_PLACEMENT_3D ( 'NONE', #1517, #7341, #7384 ) ;
#7093=VERTEX_POINT ( 'NONE', #4295 ) ;
#7096=ADVANCED_FACE ( 'NONE', ( #5750 ), #5221, .F. ) ;
#7104=EDGE_CURVE ( 'NONE', #1688, #75, #6944, .T. ) ;
#7107=CARTESIAN_POINT ( 'NONE',  ( 9.998427761233271482, -32.39925913208585939, -3.252606517456513302E-14 ) ) ;
#7110=LINE ( 'NONE', #1293, #6965 ) ;
#7113=AXIS2_PLACEMENT_3D ( 'NONE', #5018, #4533, #2781 ) ;
#7114=CARTESIAN_POINT ( 'NONE',  ( 14.12411727399747186, 19.86467175049790868, 0.006154456448484880299 ) ) ;
#7116=CIRCLE ( 'NONE', #7360, 0.7499999999999896749 ) ;
#7121=B_SPLINE_CURVE_WITH_KNOTS ( 'NONE', 3,
 ( #2188, #1598, #3887, #1034 ),
 .UNSPECIFIED., .F., .F.,
 ( 4, 4 ),
 ( 0.000000000000000000, 1.000000000000000000 ),
 .UNSPECIFIED. ) ;
#7123=VECTOR ( 'NONE', #4247, 1000.000000000000000 ) ;
#7127=ORIENTED_EDGE ( 'NONE', *, *, #1546, .T. ) ;
#7133=CARTESIAN_POINT ( 'NONE',  ( 12.15447797363371052, 11.01039466689934798, -3.299999999999988720 ) ) ;
#7137=VECTOR ( 'NONE', #720, 1000.000000000000114 ) ;
#7138=EDGE_LOOP ( 'NONE', ( #1154, #900, #6034, #1078 ) ) ;
#7140=LINE ( 'NONE', #2510, #7123 ) ;
#7141=LINE ( 'NONE', #3103, #660 ) ;
#7143=DIRECTION ( 'NONE',  ( -5.715354789845005112E-18, -9.999836672264339449E-16, 1.000000000000000000 ) ) ;
#7150=FACE_OUTER_BOUND ( 'NONE', #4093, .T. ) ;
#7155=CARTESIAN_POINT ( 'NONE',  ( 22.42915535073480982, 21.39736943723329432, -1.493845543551513444 ) ) ;
#7161=DIRECTION ( 'NONE',  ( 0.4039838799357093335, 0.9147661038495527031, 1.550530988647994607E-16 ) ) ;
#7164=ORIENTED_EDGE ( 'NONE', *, *, #4334, .F. ) ;
#7165=ORIENTED_EDGE ( 'NONE', *, *, #4355, .F. ) ;
#7170=DIRECTION ( 'NONE',  ( 5.715354789845005112E-18, 9.999836672264339449E-16, -1.000000000000000000 ) ) ;
#7172=VERTEX_POINT ( 'NONE', #2352 ) ;
#7177=DIRECTION ( 'NONE',  ( -5.715354789845005112E-18, -9.999836672264339449E-16, 1.000000000000000000 ) ) ;
#7186=ORIENTED_EDGE ( 'NONE', *, *, #104, .T. ) ;
#7187=CARTESIAN_POINT ( 'NONE',  ( 1.714606436953501688E-17, 2.999951001679301835E-15, 0.000000000000000000 ) ) ;
#7189=ORIENTED_EDGE ( 'NONE', *, *, #198, .F. ) ;
#7192=DIRECTION ( 'NONE',  ( 0.3213584079436493934, -0.3547505615521249767, 0.8779981849197495691 ) ) ;
#7196=PLANE ( 'NONE',  #1737 ) ;
#7198=DIRECTION ( 'NONE',  ( -5.715354789845005112E-18, -9.999836672264339449E-16, 1.000000000000000000 ) ) ;
#7200=ORIENTED_EDGE ( 'NONE', *, *, #1780, .T. ) ;
#7205=CARTESIAN_POINT ( 'NONE',  ( 8.042591699913112180, 16.36558300704127689, 1.647987302177966740E-14 ) ) ;
#7207=CARTESIAN_POINT ( 'NONE',  ( 41.70778007397900211, -94.98992620957551480, -9.454242944073598665E-14 ) ) ;
#7209=ORIENTED_EDGE ( 'NONE', *, *, #1448, .T. ) ;
#7214=CARTESIAN_POINT ( 'NONE',  ( -20.16480223318149356, 14.61937842657788167, 0.006154456448479242447 ) ) ;
#7222=VECTOR ( 'NONE', #4053, 1000.000000000000227 ) ;
#7226=VECTOR ( 'NONE', #950, 1000.000000000000114 ) ;
#7228=ORIENTED_EDGE ( 'NONE', *, *, #5854, .T. ) ;
#7229=LINE ( 'NONE', #6224, #3891 ) ;
#7234=ADVANCED_FACE ( 'NONE', ( #2101 ), #1542, .F. ) ;
#7236=AXIS2_PLACEMENT_3D ( 'NONE', #5435, #5396, #5973 ) ;
#7238=AXIS2_PLACEMENT_3D ( 'NONE', #4476, #1647, #5619 ) ;
#7239=CARTESIAN_POINT ( 'NONE',  ( 15.39542127499540136, -35.83857563806657964, -3.556183125752454544E-14 ) ) ;
#7240=DIRECTION ( 'NONE',  ( 0.3963837160139272453, 0.9180849359830441925, 9.203354146796070219E-16 ) ) ;
#7244=CARTESIAN_POINT ( 'NONE',  ( -3.749938752099124972, 0.02143258046192221891, 0.000000000000000000 ) ) ;
#7248=ORIENTED_EDGE ( 'NONE', *, *, #1200, .F. ) ;
#7249=CIRCLE ( 'NONE', #5946, 0.7500000000000003331 ) ;
#7257=CARTESIAN_POINT ( 'NONE',  ( 43.95774332523846795, -95.00278575785266355, -9.454242944073598665E-14 ) ) ;
#7260=CIRCLE ( 'NONE', #7238, 0.7499999999999872324 ) ;
#7263=CONICAL_SURFACE ( 'NONE', #4641, 0.7499999999999872324, 1.029744258676647872 ) ;
#7265=DIRECTION ( 'NONE',  ( 5.715354789845005112E-18, 9.999836672264339449E-16, -1.000000000000000000 ) ) ;
#7267=FACE_OUTER_BOUND ( 'NONE', #809, .T. ) ;
#7268=DIRECTION ( 'NONE',  ( -0.6713653717953991240, 0.7411265327553895332, 8.112475779533124710E-16 ) ) ;
#7273=DIRECTION ( 'NONE',  ( -5.715354789845005112E-18, -9.999836672264339449E-16, 1.000000000000000000 ) ) ;
#7274=ADVANCED_FACE ( 'NONE', ( #6619 ), #2667, .T. ) ;
#7276=DIRECTION ( 'NONE',  ( -0.9999836672264333925, 0.005715354789844388425, 0.000000000000000000 ) ) ;
#7278=CARTESIAN_POINT ( 'NONE',  ( 27.65533861039806496, -36.12687000486608468, 2.999999999999964029 ) ) ;
#7282=ORIENTED_EDGE ( 'NONE', *, *, #6655, .T. ) ;
#7283=VERTEX_POINT ( 'NONE', #3262 ) ;
#7284=EDGE_CURVE ( 'NONE', #2912, #553, #5582, .T. ) ;
#7287=CARTESIAN_POINT ( 'NONE',  ( -20.16480223318149356, 14.61937842657788345, -2.993845543551524990 ) ) ;
#7289=CARTESIAN_POINT ( 'NONE',  ( 12.15447797363371052, 11.01039466689934443, 1.127570259384924611E-14 ) ) ;
#7293=LINE ( 'NONE', #1651, #4964 ) ;
#7294=DIRECTION ( 'NONE',  ( 5.715354789845005112E-18, 9.999836672264339449E-16, -1.000000000000000000 ) ) ;
#7297=ORIENTED_EDGE ( 'NONE', *, *, #6919, .T. ) ;
#7298=DIRECTION ( 'NONE',  ( 0.6713653717953966815, -0.7411265327553919757, -7.372773368101216216E-16 ) ) ;
#7299=LINE ( 'NONE', #3913, #3240 ) ;
#7300=ORIENTED_EDGE ( 'NONE', *, *, #7416, .T. ) ;
#7301=ADVANCED_FACE ( 'NONE', ( #337 ), #3753, .T. ) ;
#7303=DIRECTION ( 'NONE',  ( -5.715354789845005112E-18, -9.999836672264339449E-16, 1.000000000000000000 ) ) ;
#7304=CARTESIAN_POINT ( 'NONE',  ( 24.99346688245966419, 26.01411140189437532, -2.993845543551503674 ) ) ;
#7306=DIRECTION ( 'NONE',  ( -0.9147661038495519259, 0.4039838799357108878, 4.130293990420968897E-16 ) ) ;
#7308=CARTESIAN_POINT ( 'NONE',  ( 12.40979888490706706, -30.61452125107580713, -3.035766082959412415E-14 ) ) ;
#7311=DIRECTION ( 'NONE',  ( 0.9999836672264332815, -0.005715354789845002517, 0.000000000000000000 ) ) ;
#7314=DIRECTION ( 'NONE',  ( -3.347047707994206215E-17, -9.998250342643943298E-16, 1.000000000000000000 ) ) ;
#7316=EDGE_CURVE ( 'NONE', #212, #5062, #5334, .T. ) ;
#7317=VERTEX_POINT ( 'NONE', #3306 ) ;
#7320=CARTESIAN_POINT ( 'NONE',  ( -11.31173072208887831, -97.70380408000731620, -9.757819552369539906E-14 ) ) ;
#7321=ORIENTED_EDGE ( 'NONE', *, *, #3659, .T. ) ;
#7324=DIRECTION ( 'NONE',  ( 5.715354789845005112E-18, 9.999836672264339449E-16, -1.000000000000000000 ) ) ;
#7334=CARTESIAN_POINT ( 'NONE',  ( 39.97800414936823188, -95.26063634933134949, 2.999999999999904965 ) ) ;
#7335=LINE ( 'NONE', #6119, #2524 ) ;
#7336=ADVANCED_FACE ( 'NONE', ( #35 ), #3226, .F. ) ;
#7341=DIRECTION ( 'NONE',  ( 5.715354789845005112E-18, 9.999836672264339449E-16, -1.000000000000000000 ) ) ;
#7343=DIRECTION ( 'NONE',  ( 0.6713653717953970146, -0.7411265327553913096, -7.372773368101209313E-16 ) ) ;
#7355=ORIENTED_EDGE ( 'NONE', *, *, #1427, .F. ) ;
#7356=ORIENTED_EDGE ( 'NONE', *, *, #6778, .F. ) ;
#7359=CARTESIAN_POINT ( 'NONE',  ( 15.82006518139331774, 14.33094549030129983, -2.230393353321895145 ) ) ;
#7360=AXIS2_PLACEMENT_3D ( 'NONE', #5694, #1136, #2367 ) ;
#7361=EDGE_CURVE ( 'NONE', #3666, #3563, #7116, .T. ) ;
#7363=DIRECTION ( 'NONE',  ( -0.6713653717954000122, 0.7411265327553888671, 8.673617379884183383E-16 ) ) ;
#7365=VECTOR ( 'NONE', #1201, 1000.000000000000227 ) ;
#7369=DIRECTION ( 'NONE',  ( 0.7411265327553895332, 0.6713653717953992350, 6.755902076156661002E-16 ) ) ;
#7371=VECTOR ( 'NONE', #6977, 1000.000000000000000 ) ;
#7373=DIRECTION ( 'NONE',  ( -5.715354789845005112E-18, -9.999836672264339449E-16, 1.000000000000000000 ) ) ;
#7374=CIRCLE ( 'NONE', #4138, 3.300000000000000711 ) ;
#7377=CARTESIAN_POINT ( 'NONE',  ( 39.97800414936823188, -95.26063634933134949, -3.001370543551635794 ) ) ;
#7383=CARTESIAN_POINT ( 'NONE',  ( -16.44258018226587836, 7.261459853215404436, -0.3999035282155121718 ) ) ;
#7384=DIRECTION ( 'NONE',  ( 0.9999836672264332815, -0.005715354789845002517, 0.000000000000000000 ) ) ;
#7387=CARTESIAN_POINT ( 'NONE',  ( 43.89994888609457035, -93.87291691326068133, 2.999999999999906297 ) ) ;
#7388=ORIENTED_EDGE ( 'NONE', *, *, #5784, .F. ) ;
#7389=CARTESIAN_POINT ( 'NONE',  ( -20.16480223318149356, 14.61937842657788167, 0.006154456448484012937 ) ) ;
#7391=FACE_OUTER_BOUND ( 'NONE', #3665, .T. ) ;
#7393=CARTESIAN_POINT ( 'NONE',  ( 43.45632180942044442, -94.90042465344848210, 2.999999999999905409 ) ) ;
#7399=ORIENTED_EDGE ( 'NONE', *, *, #6459, .F. ) ;
#7400=ORIENTED_EDGE ( 'NONE', *, *, #1280, .F. ) ;
#7402=ORIENTED_EDGE ( 'NONE', *, *, #5359, .T. ) ;
#7404=CARTESIAN_POINT ( 'NONE',  ( 12.15447797363371052, 11.01039466689934798, -3.299999999999988720 ) ) ;
#7406=ORIENTED_EDGE ( 'NONE', *, *, #5712, .T. ) ;
#7407=ORIENTED_EDGE ( 'NONE', *, *, #5919, .F. ) ;
#7416=EDGE_CURVE ( 'NONE', #7431, #6609, #2187, .T. ) ;
#7419=DIRECTION ( 'NONE',  ( -5.715354789845005112E-18, -9.999836672264339449E-16, 1.000000000000000000 ) ) ;
#7425=DIRECTION ( 'NONE',  ( 5.715354789845005112E-18, 9.999836672264339449E-16, -1.000000000000000000 ) ) ;
#7427=LINE ( 'NONE', #4050, #6304 ) ;
#7431=VERTEX_POINT ( 'NONE', #2254 ) ;
#7432=ADVANCED_FACE ( 'NONE', ( #6929 ), #3986, .T. ) ;
#7433=EDGE_LOOP ( 'NONE', ( #5166, #2619 ) ) ;
#7434=VERTEX_POINT ( 'NONE', #1208 ) ;
#7438=DIRECTION ( 'NONE',  ( 0.5818022356294096920, -0.8133302887613499399, -8.099917986277619058E-16 ) ) ;
#7439=FACE_OUTER_BOUND ( 'NONE', #559, .T. ) ;
ENDSEC;
END-ISO-10303-21;
